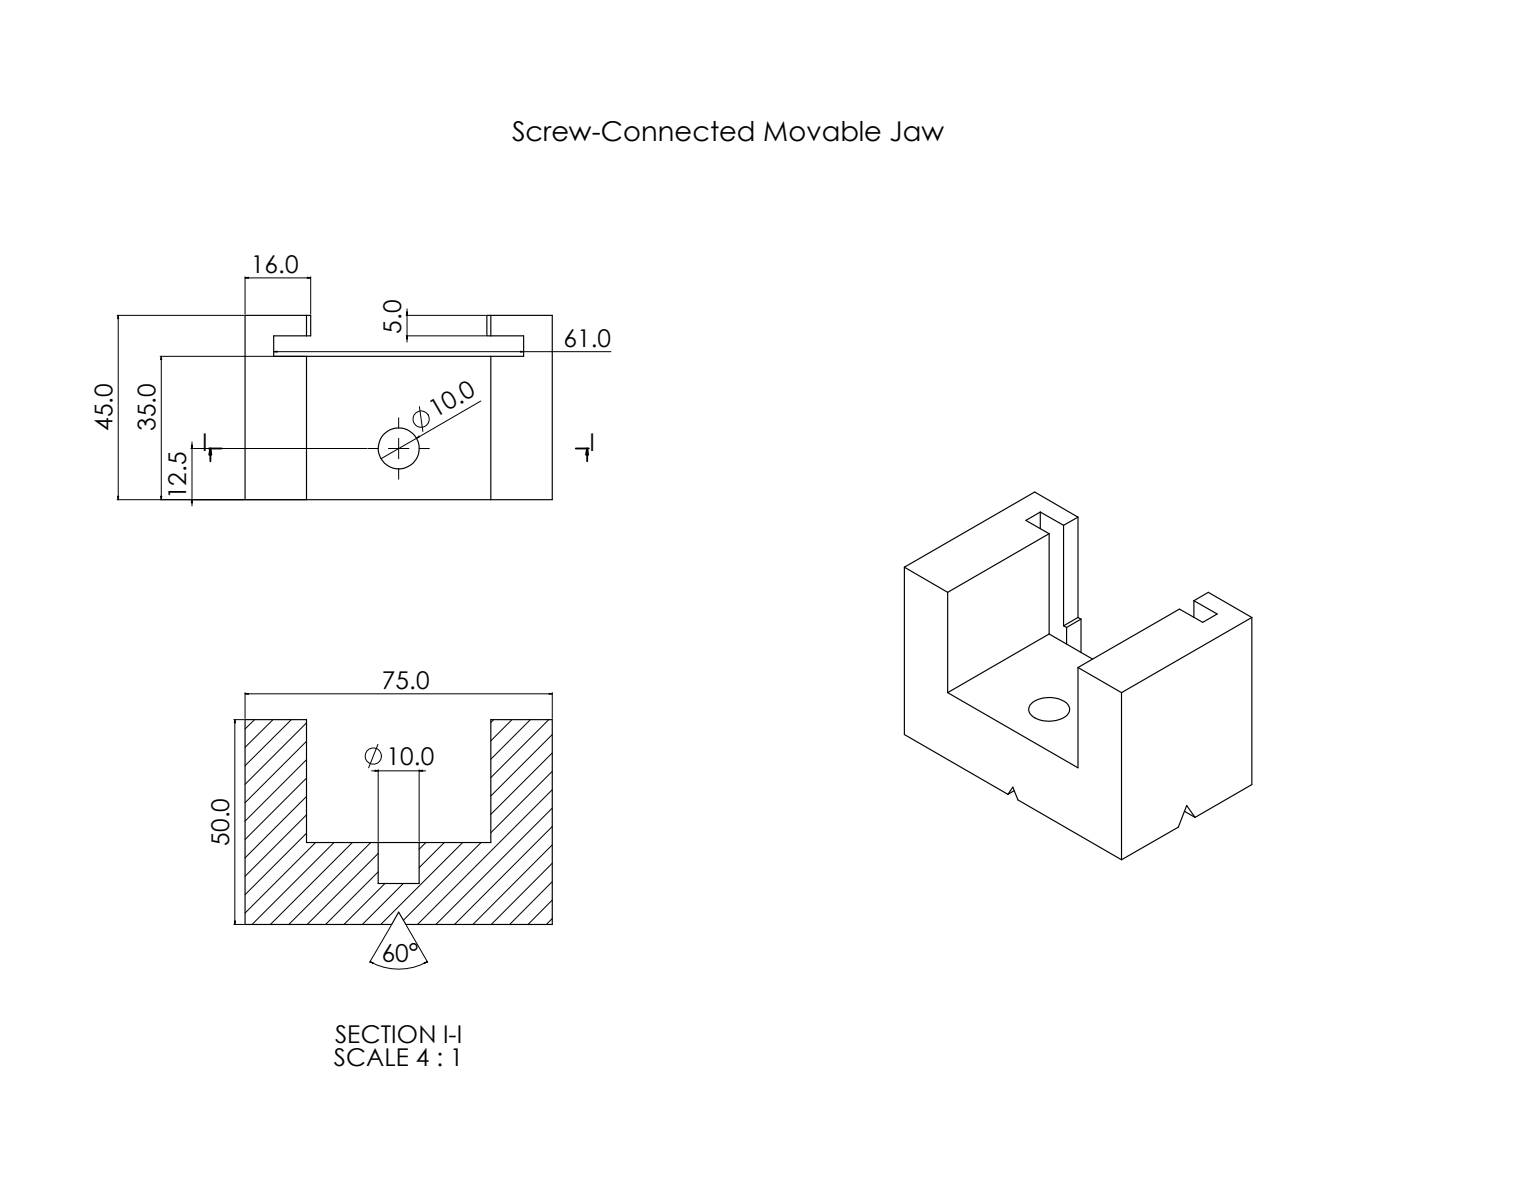
ISO-10303-21;
HEADER;
FILE_DESCRIPTION (('STEP AP214'),
    '1' );
FILE_NAME ('Screw-Connected Movable Jaw.step',
    '2026-10-24T22:31:37',
    ( '' ),
    ( '' ),
    'SwSTEP 2.0',
    'SolidWorks 2025',
    '' );
FILE_SCHEMA (( 'AUTOMOTIVE_DESIGN' ));
ENDSEC;

DATA;
#62=DIRECTION ( 'NONE',  ( 0.000000000000000000, -1.000000000000000000, 1.090355031989287297E-16 ) ) ;
#117=LINE ( 'NONE', #62385, #16927 ) ;
#143=CARTESIAN_POINT ( 'NONE',  ( -37.33262083840156009, 163.6868197944959888, -1.732050807568741524 ) ) ;
#194=ORIENTED_EDGE ( 'NONE', *, *, #7075, .T. ) ;
#425=EDGE_CURVE ( 'NONE', #74638, #6038, #70695, .T. ) ;
#505=DIRECTION ( 'NONE',  ( -0.8660254037844385966, -0.4999999999999999445, 5.782411586589351229E-17 ) ) ;
#555=DIRECTION ( 'NONE',  ( -0.8660254037844384856, -0.5000000000000002220, 5.782411586589354927E-17 ) ) ;
#594=ORIENTED_EDGE ( 'NONE', *, *, #77639, .T. ) ;
#731=ADVANCED_FACE ( 'NONE', ( #78063 ), #54223, .F. ) ;
#750=CARTESIAN_POINT ( 'NONE',  ( -17.69472717286124208, 126.6729902121449811, 2.598076211353400389 ) ) ;
#879=EDGE_CURVE ( 'NONE', #47755, #61485, #20257, .T. ) ;
#908=CARTESIAN_POINT ( 'NONE',  ( 5.968649350820379063, 188.6868197944959604, -22.49999999999984368 ) ) ;
#1042=ADVANCED_FACE ( 'NONE', ( #29840 ), #14643, .F. ) ;
#1055=DIRECTION ( 'NONE',  ( 3.817860598523670672E-18, 1.090355031989287297E-16, 1.000000000000000000 ) ) ;
#1129=ORIENTED_EDGE ( 'NONE', *, *, #70913, .F. ) ;
#1239=DIRECTION ( 'NONE',  ( 0.5000000000000004441, -0.8660254037844383745, -0.000000000000000000 ) ) ;
#1415=LINE ( 'NONE', #87069, #9047 ) ;
#1497=EDGE_LOOP ( 'NONE', ( #50090, #79860, #594, #87888 ) ) ;
#1639=EDGE_CURVE ( 'NONE', #18415, #51452, #44648, .T. ) ;
#2048=EDGE_CURVE ( 'NONE', #72912, #83865, #78409, .T. ) ;
#2098=ORIENTED_EDGE ( 'NONE', *, *, #49119, .T. ) ;
#2149=LINE ( 'NONE', #78150, #15677 ) ;
#2199=CLOSED_SHELL ( 'NONE', ( #75150, #7233, #84553, #37271, #22213, #44129, #61711, #25953, #74022, #4386, #1042, #68700, #27934, #56439, #64130, #11572, #38638, #98679, #79121, #731, #36244, #12582, #9749, #91004, #12653, #26400, #28305, #79766, #19607, #61517, #59063, #68707, #71578, #39382 ) ) ;
#2227=PRODUCT_DEFINITION_SHAPE ( 'NONE', 'NONE',  #80010 ) ;
#2485=ORIENTED_EDGE ( 'NONE', *, *, #31531, .F. ) ;
#2498=CARTESIAN_POINT ( 'NONE',  ( 5.968649350820482979, 188.6868197944959320, -37.49999999999994316 ) ) ;
#2564=ORIENTED_EDGE ( 'NONE', *, *, #90628, .T. ) ;
#2631=VECTOR ( 'NONE', #64054, 1000.000000000000000 ) ;
#2646=EDGE_CURVE ( 'NONE', #86838, #32226, #4151, .T. ) ;
#2647=CARTESIAN_POINT ( 'NONE',  ( -41.79694972978692391, 146.7012482093458914, -8.867527416774462878 ) ) ;
#2969=CARTESIAN_POINT ( 'NONE',  ( 2.487887237287232711, 134.7156766241960497, 22.50000000000002132 ) ) ;
#3041=VECTOR ( 'NONE', #9744, 1000.000000000000114 ) ;
#3155=ORIENTED_EDGE ( 'NONE', *, *, #18849, .T. ) ;
#3325=EDGE_LOOP ( 'NONE', ( #87906, #41347, #44835, #33520 ) ) ;
#3401=LINE ( 'NONE', #96620, #5789 ) ;
#3471=EDGE_CURVE ( 'NONE', #73274, #82623, #43663, .T. ) ;
#3574=CARTESIAN_POINT ( 'NONE',  ( -22.42236680055716036, 157.8615022471903444, 5.188172501216621122E-14 ) ) ;
#3633=CARTESIAN_POINT ( 'NONE',  ( -14.83262083840143575, 124.7156766241961208, 21.50000000000006750 ) ) ;
#3874=DIRECTION ( 'NONE',  ( -0.8660254037844384856, -0.5000000000000002220, -3.252519625699449945E-16 ) ) ;
#4014=LINE ( 'NONE', #33416, #90354 ) ;
#4047=LINE ( 'NONE', #87232, #75251 ) ;
#4062=ORIENTED_EDGE ( 'NONE', *, *, #77189, .T. ) ;
#4065=CARTESIAN_POINT ( 'NONE',  ( -14.83262083840142154, 124.7156766241961208, -37.49999999999995737 ) ) ;
#4151=LINE ( 'NONE', #80716, #24806 ) ;
#4181=CARTESIAN_POINT ( 'NONE',  ( -26.08262083840154233, 139.2012482093457493, 37.49999999999996447 ) ) ;
#4349=VERTEX_POINT ( 'NONE', #79754 ) ;
#4386=ADVANCED_FACE ( 'NONE', ( #59755 ), #36460, .F. ) ;
#4388=VECTOR ( 'NONE', #14547, 1000.000000000000000 ) ;
#4548=DIRECTION ( 'NONE',  ( -0.5000000000000003331, 0.8660254037844383745, 0.000000000000000000 ) ) ;
#4553=LINE ( 'NONE', #50644, #84057 ) ;
#4562=EDGE_CURVE ( 'NONE', #63766, #16186, #49551, .T. ) ;
#4738=FACE_OUTER_BOUND ( 'NONE', #58855, .T. ) ;
#4995=LINE ( 'NONE', #28269, #80233 ) ;
#5582=EDGE_CURVE ( 'NONE', #6163, #74234, #97394, .T. ) ;
#5666=VERTEX_POINT ( 'NONE', #10167 ) ;
#5677=ORIENTED_EDGE ( 'NONE', *, *, #59489, .F. ) ;
#5789=VECTOR ( 'NONE', #57061, 1000.000000000000000 ) ;
#5914=ORIENTED_EDGE ( 'NONE', *, *, #17435, .T. ) ;
#6038=VERTEX_POINT ( 'NONE', #64241 ) ;
#6163=VERTEX_POINT ( 'NONE', #89116 ) ;
#6186=VECTOR ( 'NONE', #3874, 1000.000000000000227 ) ;
#6215=EDGE_LOOP ( 'NONE', ( #59856, #62245, #86227, #58381 ) ) ;
#6329=CARTESIAN_POINT ( 'NONE',  ( -13.79761285583127872, 128.9229902121449811, 8.559299291603829198E-14 ) ) ;
#6632=VECTOR ( 'NONE', #76579, 1000.000000000000000 ) ;
#6865=DIRECTION ( 'NONE',  ( -2.168404344971021440E-16, 3.755786496842916807E-16, 1.000000000000000000 ) ) ;
#7006=VECTOR ( 'NONE', #78316, 1000.000000000000227 ) ;
#7075=EDGE_CURVE ( 'NONE', #88359, #90349, #41118, .T. ) ;
#7233=ADVANCED_FACE ( 'NONE', ( #82682 ), #51213, .F. ) ;
#7251=CARTESIAN_POINT ( 'NONE',  ( -17.33262083840142509, 129.0458036431182904, -30.52142883766501669 ) ) ;
#7266=CARTESIAN_POINT ( 'NONE',  ( -20.01211276271284945, 173.6868197944959036, -22.49999999999984013 ) ) ;
#7563=CARTESIAN_POINT ( 'NONE',  ( -19.83262083840137180, 133.3759306620404459, -30.52142883766495629 ) ) ;
#7571=SHAPE_REPRESENTATION ( 'Screw-Connected Movable Jaw', ( #68784 ), #31602 ) ;
#7578=VERTEX_POINT ( 'NONE', #71701 ) ;
#7683=CARTESIAN_POINT ( 'NONE',  ( -2.512112762712735314, 143.3759306620403891, -22.49999999999983658 ) ) ;
#7854=VECTOR ( 'NONE', #27344, 1000.000000000000000 ) ;
#7870=CARTESIAN_POINT ( 'NONE',  ( -37.33262083840156720, 163.6868197944959888, 1.732050807568908724 ) ) ;
#7916=DIRECTION ( 'NONE',  ( -0.5000000000000001110, 0.8660254037844384856, 0.000000000000000000 ) ) ;
#8114=LINE ( 'NONE', #22304, #30135 ) ;
#8168=ORIENTED_EDGE ( 'NONE', *, *, #19129, .T. ) ;
#8212=CARTESIAN_POINT ( 'NONE',  ( 28.46864935082050252, 149.7156766241961350, -37.49999999999994316 ) ) ;
#8322=VERTEX_POINT ( 'NONE', #70686 ) ;
#8363=PLANE ( 'NONE',  #70920 ) ;
#8478=EDGE_LOOP ( 'NONE', ( #51154, #77489, #24724, #33114, #10678, #81299 ) ) ;
#8670=EDGE_LOOP ( 'NONE', ( #87000, #21456, #59012, #82999, #14658, #48072, #24313, #5677 ) ) ;
#8671=ORIENTED_EDGE ( 'NONE', *, *, #77189, .F. ) ;
#8776=VERTEX_POINT ( 'NONE', #83914 ) ;
#8850=UNCERTAINTY_MEASURE_WITH_UNIT (LENGTH_MEASURE( 1.000000000000000082E-05 ), #27316, 'distance_accuracy_value', 'NONE');
#8993=CARTESIAN_POINT ( 'NONE',  ( -0.01211276271276783001, 139.0458036431182620, -22.49999999999983658 ) ) ;
#9045=ORIENTED_EDGE ( 'NONE', *, *, #14029, .T. ) ;
#9047=VECTOR ( 'NONE', #11022, 1000.000000000000000 ) ;
#9248=VECTOR ( 'NONE', #40481, 1000.000000000000114 ) ;
#9460=ORIENTED_EDGE ( 'NONE', *, *, #61819, .F. ) ;
#9580=CARTESIAN_POINT ( 'NONE',  ( -14.83262083840143575, 124.7156766241961208, -21.50000000000003197 ) ) ;
#9618=CARTESIAN_POINT ( 'NONE',  ( 19.98788723728717898, 104.4047874917408336, 22.50000000000002132 ) ) ;
#9744=DIRECTION ( 'NONE',  ( 0.5000000000000004441, -0.8660254037844383745, -0.000000000000000000 ) ) ;
#9749=ADVANCED_FACE ( 'NONE', ( #58583 ), #19135, .F. ) ;
#9823=CARTESIAN_POINT ( 'NONE',  ( 5.968649350820482979, 188.6868197944959320, -37.49999999999994316 ) ) ;
#9826=ORIENTED_EDGE ( 'NONE', *, *, #15394, .F. ) ;
#9889=ORIENTED_EDGE ( 'NONE', *, *, #15394, .T. ) ;
#9934=ORIENTED_EDGE ( 'NONE', *, *, #92492, .F. ) ;
#9947=EDGE_CURVE ( 'NONE', #12823, #82885, #37288, .T. ) ;
#9975=VECTOR ( 'NONE', #45768, 1000.000000000000000 ) ;
#9992=LINE ( 'NONE', #32770, #17278 ) ;
#10061=ORIENTED_EDGE ( 'NONE', *, *, #19856, .T. ) ;
#10167=CARTESIAN_POINT ( 'NONE',  ( -17.33262083840143930, 129.0458036431182904, 21.50000000000006750 ) ) ;
#10240=DIRECTION ( 'NONE',  ( -0.8944271909999158554, 0.000000000000000000, -0.4472135954999578722 ) ) ;
#10434=ORIENTED_EDGE ( 'NONE', *, *, #88822, .F. ) ;
#10616=ORIENTED_EDGE ( 'NONE', *, *, #56292, .F. ) ;
#10634=ORIENTED_EDGE ( 'NONE', *, *, #76967, .F. ) ;
#10642=LINE ( 'NONE', #71447, #37753 ) ;
#10678=ORIENTED_EDGE ( 'NONE', *, *, #71015, .T. ) ;
#10704=VECTOR ( 'NONE', #12962, 1000.000000000000227 ) ;
#10811=LINE ( 'NONE', #9823, #16722 ) ;
#10925=AXIS2_PLACEMENT_3D ( 'NONE', #55046, #78378, #18578 ) ;
#11022=DIRECTION ( 'NONE',  ( 0.8660254037844384856, 0.5000000000000002220, -5.782411586589354927E-17 ) ) ;
#11049=AXIS2_PLACEMENT_3D ( 'NONE', #65578, #50871, #42267 ) ;
#11078=CARTESIAN_POINT ( 'NONE',  ( 86.18027666378026197, 49.75620593066997799, 22.50000000000002842 ) ) ;
#11080=CARTESIAN_POINT ( 'NONE',  ( 42.87900647455834502, 24.75620593066997444, 1.732050807568941364 ) ) ;
#11087=CARTESIAN_POINT ( 'NONE',  ( 23.46864935082055581, 158.3759306620404743, -30.52142883766493853 ) ) ;
#11207=AXIS2_PLACEMENT_3D ( 'NONE', #41992, #58187, #72929 ) ;
#11363=ORIENTED_EDGE ( 'NONE', *, *, #96502, .F. ) ;
#11572=ADVANCED_FACE ( 'NONE', ( #50894 ), #27119, .F. ) ;
#11625=CARTESIAN_POINT ( 'NONE',  ( -11.26211276271278194, 158.5313752282681605, 5.249404841173988696E-14 ) ) ;
#11665=ORIENTED_EDGE ( 'NONE', *, *, #5582, .F. ) ;
#11880=PLANE ( 'NONE',  #54755 ) ;
#11930=PLANE ( 'NONE',  #43280 ) ;
#12162=FACE_OUTER_BOUND ( 'NONE', #51047, .T. ) ;
#12401=EDGE_CURVE ( 'NONE', #47755, #60445, #37275, .T. ) ;
#12582=ADVANCED_FACE ( 'NONE', ( #48381 ), #79325, .F. ) ;
#12653=ADVANCED_FACE ( 'NONE', ( #47118 ), #78039, .F. ) ;
#12667=CARTESIAN_POINT ( 'NONE',  ( -2.631798339875063064, 146.7012482093458914, -10.71504827818132277 ) ) ;
#12669=LINE ( 'NONE', #50636, #79981 ) ;
#12690=DIRECTION ( 'NONE',  ( 0.5000000000000004441, -0.8660254037844383745, -0.000000000000000000 ) ) ;
#12819=ORIENTED_EDGE ( 'NONE', *, *, #22660, .F. ) ;
#12823=VERTEX_POINT ( 'NONE', #96261 ) ;
#12846=CARTESIAN_POINT ( 'NONE',  ( -17.23454462704816947, 134.8759306620403038, 8.559299000364187034E-14 ) ) ;
#12962=DIRECTION ( 'NONE',  ( -0.8660254037844384856, -0.5000000000000002220, -3.252519625699449945E-16 ) ) ;
#13026=CARTESIAN_POINT ( 'NONE',  ( 25.96864935082048831, 154.0458036431183189, 30.52142883766506998 ) ) ;
#13092=VECTOR ( 'NONE', #72623, 1000.000000000000114 ) ;
#13113=FACE_OUTER_BOUND ( 'NONE', #15810, .T. ) ;
#13355=VECTOR ( 'NONE', #1239, 1000.000000000000114 ) ;
#13424=DIRECTION ( 'NONE',  ( 0.000000000000000000, 1.000000000000000000, 1.097929109219269329E-14 ) ) ;
#13577=FACE_OUTER_BOUND ( 'NONE', #6215, .T. ) ;
#13610=LINE ( 'NONE', #92150, #40083 ) ;
#13623=VECTOR ( 'NONE', #34224, 1000.000000000000114 ) ;
#13774=EDGE_LOOP ( 'NONE', ( #73707, #8671, #89866, #94192, #87422, #20562, #50702 ) ) ;
#13881=ORIENTED_EDGE ( 'NONE', *, *, #31531, .T. ) ;
#14029=EDGE_CURVE ( 'NONE', #61860, #89848, #10642, .T. ) ;
#14037=VECTOR ( 'NONE', #96964, 1000.000000000000227 ) ;
#14064=DIRECTION ( 'NONE',  ( -0.8944271909999158554, 0.000000000000000000, -0.4472135954999578722 ) ) ;
#14371=CARTESIAN_POINT ( 'NONE',  ( -21.75249381947928740, 146.7012482093458914, -37.49999999999995737 ) ) ;
#14434=DIRECTION ( 'NONE',  ( -0.5000000000000003331, 0.8660254037844383745, -9.251858538542982674E-17 ) ) ;
#14515=CARTESIAN_POINT ( 'NONE',  ( 86.18027666378027618, 49.75620593066998509, 1.003037947553365612E-13 ) ) ;
#14526=VERTEX_POINT ( 'NONE', #77303 ) ;
#14547=DIRECTION ( 'NONE',  ( -0.000000000000000000, -0.000000000000000000, 1.000000000000000000 ) ) ;
#14601=CARTESIAN_POINT ( 'NONE',  ( -13.79761285583127872, 128.9229902121449811, 8.559299291603829198E-14 ) ) ;
#14643=PLANE ( 'NONE',  #53793 ) ;
#14658=ORIENTED_EDGE ( 'NONE', *, *, #22404, .F. ) ;
#14688=ORIENTED_EDGE ( 'NONE', *, *, #42973, .F. ) ;
#15205=VERTEX_POINT ( 'NONE', #61955 ) ;
#15311=ORIENTED_EDGE ( 'NONE', *, *, #85316, .T. ) ;
#15354=CARTESIAN_POINT ( 'NONE',  ( 0.000000000000000000, 0.000000000000000000, 0.000000000000000000 ) ) ;
#15394=EDGE_CURVE ( 'NONE', #91009, #24841, #31779, .T. ) ;
#15543=ORIENTED_EDGE ( 'NONE', *, *, #53881, .F. ) ;
#15633=CARTESIAN_POINT ( 'NONE',  ( -21.75249381947928740, 146.7012482093458914, -48.95643923738973768 ) ) ;
#15677=VECTOR ( 'NONE', #32021, 1000.000000000000000 ) ;
#15689=DIRECTION ( 'NONE',  ( 0.8660254037844384856, 0.5000000000000002220, 0.000000000000000000 ) ) ;
#15810=EDGE_LOOP ( 'NONE', ( #17648, #1129, #54369, #36084 ) ) ;
#15951=CARTESIAN_POINT ( 'NONE',  ( 25.96864935082048831, 154.0458036431183189, 21.50000000000008527 ) ) ;
#16186=VERTEX_POINT ( 'NONE', #26218 ) ;
#16529=VERTEX_POINT ( 'NONE', #7266 ) ;
#16685=EDGE_CURVE ( 'NONE', #82885, #18415, #35514, .T. ) ;
#16722=VECTOR ( 'NONE', #65493, 1000.000000000000000 ) ;
#16908=EDGE_CURVE ( 'NONE', #6038, #8322, #9992, .T. ) ;
#16927=VECTOR ( 'NONE', #23898, 1000.000000000000227 ) ;
#17115=EDGE_CURVE ( 'NONE', #27140, #32226, #65792, .T. ) ;
#17141=VERTEX_POINT ( 'NONE', #37257 ) ;
#17278=VECTOR ( 'NONE', #31755, 999.9999999999998863 ) ;
#17419=CARTESIAN_POINT ( 'NONE',  ( -37.33262083840143930, 163.6868197944959036, -37.49999999999995737 ) ) ;
#17422=CARTESIAN_POINT ( 'NONE',  ( 5.968649350820482979, 188.6868197944959320, -37.49999999999994316 ) ) ;
#17430=ORIENTED_EDGE ( 'NONE', *, *, #98473, .F. ) ;
#17435=EDGE_CURVE ( 'NONE', #5666, #82885, #2149, .T. ) ;
#17498=VERTEX_POINT ( 'NONE', #143 ) ;
#17537=VECTOR ( 'NONE', #29031, 999.9999999999998863 ) ;
#17648=ORIENTED_EDGE ( 'NONE', *, *, #85806, .T. ) ;
#17687=VERTEX_POINT ( 'NONE', #82679 ) ;
#17710=LINE ( 'NONE', #25295, #28391 ) ;
#17920=ORIENTED_EDGE ( 'NONE', *, *, #85209, .T. ) ;
#17929=ORIENTED_EDGE ( 'NONE', *, *, #45726, .T. ) ;
#17990=DIRECTION ( 'NONE',  ( 0.000000000000000000, -1.000000000000000000, 1.090355031989287297E-16 ) ) ;
#18047=ORIENTED_EDGE ( 'NONE', *, *, #88822, .T. ) ;
#18131=CARTESIAN_POINT ( 'NONE',  ( 5.968649350820472321, 188.6868197944958752, 22.50000000000001421 ) ) ;
#18261=EDGE_CURVE ( 'NONE', #48830, #17141, #80171, .T. ) ;
#18415=VERTEX_POINT ( 'NONE', #83535 ) ;
#18479=CARTESIAN_POINT ( 'NONE',  ( 28.46864935082048831, 149.7156766241961350, -21.50000000000001421 ) ) ;
#18536=CARTESIAN_POINT ( 'NONE',  ( 2.487887237287232711, 134.7156766241960497, 21.50000000000007461 ) ) ;
#18571=CARTESIAN_POINT ( 'NONE',  ( 2.487887237287232711, 134.7156766241960497, -22.49999999999983302 ) ) ;
#18578=DIRECTION ( 'NONE',  ( 0.5000000000000003331, -0.8660254037844383745, 0.000000000000000000 ) ) ;
#18634=CARTESIAN_POINT ( 'NONE',  ( -2.512112762712737091, 143.3759306620403891, -30.52142883766493853 ) ) ;
#18664=DIRECTION ( 'NONE',  ( -2.816764622163176999E-16, -1.626259812849725466E-16, 1.000000000000000000 ) ) ;
#18849=EDGE_CURVE ( 'NONE', #65623, #88359, #32544, .T. ) ;
#18903=FACE_OUTER_BOUND ( 'NONE', #1497, .T. ) ;
#19036=( GEOMETRIC_REPRESENTATION_CONTEXT ( 3 ) GLOBAL_UNCERTAINTY_ASSIGNED_CONTEXT ( ( #8850 ) ) GLOBAL_UNIT_ASSIGNED_CONTEXT ( ( #27316, #62931, #40116 ) ) REPRESENTATION_CONTEXT ( 'NONE', 'WORKASPACE' ) );
#19049=ORIENTED_EDGE ( 'NONE', *, *, #91374, .F. ) ;
#19129=EDGE_CURVE ( 'NONE', #31218, #65623, #68910, .T. ) ;
#19135=PLANE ( 'NONE',  #98371 ) ;
#19240=VECTOR ( 'NONE', #80991, 1000.000000000000000 ) ;
#19341=CARTESIAN_POINT ( 'NONE',  ( 86.18027666378026197, 49.75620593066997799, 22.50000000000002842 ) ) ;
#19380=AXIS2_PLACEMENT_3D ( 'NONE', #15951, #39721, #77776 ) ;
#19520=AXIS2_PLACEMENT_3D ( 'NONE', #27495, #50765, #58364 ) ;
#19582=PLANE ( 'NONE',  #49676 ) ;
#19607=ADVANCED_FACE ( 'NONE', ( #97729 ), #43986, .F. ) ;
#19629=EDGE_CURVE ( 'NONE', #63672, #16186, #1415, .T. ) ;
#19772=VECTOR ( 'NONE', #58847, 1000.000000000000114 ) ;
#19856=EDGE_CURVE ( 'NONE', #48417, #92799, #90032, .T. ) ;
#19998=VECTOR ( 'NONE', #80244, 1000.000000000000000 ) ;
#20055=DIRECTION ( 'NONE',  ( -1.000000000000000000, 0.000000000000000000, -2.816764622163176999E-16 ) ) ;
#20145=VERTEX_POINT ( 'NONE', #14371 ) ;
#20257=LINE ( 'NONE', #12667, #24876 ) ;
#20298=DIRECTION ( 'NONE',  ( 0.8660254037844385966, 0.5000000000000002220, 7.511572993685832627E-16 ) ) ;
#20423=ORIENTED_EDGE ( 'NONE', *, *, #20676, .F. ) ;
#20510=EDGE_LOOP ( 'NONE', ( #12819, #50067, #64992, #25275, #70880, #10061 ) ) ;
#20548=ORIENTED_EDGE ( 'NONE', *, *, #88172, .F. ) ;
#20562=ORIENTED_EDGE ( 'NONE', *, *, #39641, .F. ) ;
#20676=EDGE_CURVE ( 'NONE', #12823, #89585, #37230, .T. ) ;
#20793=VECTOR ( 'NONE', #95392, 1000.000000000000114 ) ;
#20803=CARTESIAN_POINT ( 'NONE',  ( 42.87900647455834502, 24.75620593066997444, 8.404119662683931360E-14 ) ) ;
#20833=DIRECTION ( 'NONE',  ( 8.673617379884076887E-16, 0.000000000000000000, -1.000000000000000000 ) ) ;
#21031=CARTESIAN_POINT ( 'NONE',  ( 25.96864935082050252, 154.0458036431183189, -30.52142883766499892 ) ) ;
#21035=AXIS2_PLACEMENT_3D ( 'NONE', #73746, #88011, #20055 ) ;
#21094=ORIENTED_EDGE ( 'NONE', *, *, #24594, .F. ) ;
#21167=DIRECTION ( 'NONE',  ( -0.8660254037844384856, -0.5000000000000002220, -3.252519625699449945E-16 ) ) ;
#21213=EDGE_CURVE ( 'NONE', #63766, #7578, #97327, .T. ) ;
#21281=DIRECTION ( 'NONE',  ( -0.5000000000000003331, 0.8660254037844385966, -4.336808689942041895E-16 ) ) ;
#21288=ORIENTED_EDGE ( 'NONE', *, *, #35737, .F. ) ;
#21324=EDGE_CURVE ( 'NONE', #70724, #90349, #4995, .T. ) ;
#21441=DIRECTION ( 'NONE',  ( -0.5000000000000003331, 0.8660254037844383745, -5.669937756276021476E-31 ) ) ;
#21456=ORIENTED_EDGE ( 'NONE', *, *, #50443, .T. ) ;
#21615=EDGE_LOOP ( 'NONE', ( #27858, #70387, #9826, #71355, #88499, #20548, #88494, #35459, #44301, #10616, #18047 ) ) ;
#21737=CARTESIAN_POINT ( 'NONE',  ( 25.96864935082050252, 154.0458036431183189, -21.50000000000001421 ) ) ;
#21741=DIRECTION ( 'NONE',  ( 1.000000000000000000, 0.000000000000000000, 2.816764622163176999E-16 ) ) ;
#21771=VERTEX_POINT ( 'NONE', #30148 ) ;
#21895=ORIENTED_EDGE ( 'NONE', *, *, #85316, .F. ) ;
#22027=DIRECTION ( 'NONE',  ( -0.4999999999999995004, 0.8660254037844389297, -1.249000902703319567E-14 ) ) ;
#22038=AXIS2_PLACEMENT_3D ( 'NONE', #74426, #88665, #73414 ) ;
#22040=EDGE_CURVE ( 'NONE', #89848, #16529, #8114, .T. ) ;
#22209=DIRECTION ( 'NONE',  ( -0.8660254037844384856, -0.5000000000000002220, 0.000000000000000000 ) ) ;
#22213=ADVANCED_FACE ( 'NONE', ( #34402 ), #90135, .T. ) ;
#22246=DIRECTION ( 'NONE',  ( -0.8660254037844384856, -0.5000000000000002220, -3.252519625699449945E-16 ) ) ;
#22304=CARTESIAN_POINT ( 'NONE',  ( 31.94941146435350987, 203.6868197944959320, -22.49999999999984368 ) ) ;
#22320=CIRCLE ( 'NONE', #95202, 4.999999999999993783 ) ;
#22347=EDGE_CURVE ( 'NONE', #49527, #70724, #55562, .T. ) ;
#22361=LINE ( 'NONE', #75088, #76135 ) ;
#22365=DIRECTION ( 'NONE',  ( 4.546899780356473057E-16, -0.000000000000000000, -1.000000000000000000 ) ) ;
#22404=EDGE_CURVE ( 'NONE', #90349, #6038, #22768, .T. ) ;
#22660=EDGE_CURVE ( 'NONE', #27862, #92799, #37221, .T. ) ;
#22768=LINE ( 'NONE', #9580, #86824 ) ;
#23037=DIRECTION ( 'NONE',  ( 0.8660254037844385966, 0.5000000000000004441, 0.000000000000000000 ) ) ;
#23066=ORIENTED_EDGE ( 'NONE', *, *, #96502, .T. ) ;
#23177=LINE ( 'NONE', #14601, #41431 ) ;
#23237=CARTESIAN_POINT ( 'NONE',  ( -24.06189489623784183, 146.7012482093458914, 8.087813781312181686E-14 ) ) ;
#23288=FACE_OUTER_BOUND ( 'NONE', #82900, .T. ) ;
#23457=DIRECTION ( 'NONE',  ( 1.000000000000000000, 0.000000000000000000, 0.000000000000000000 ) ) ;
#23898=DIRECTION ( 'NONE',  ( -0.5000000000000001110, 0.8660254037844384856, 2.775557561562890427E-17 ) ) ;
#23936=EDGE_CURVE ( 'NONE', #6163, #47559, #49559, .T. ) ;
#24052=DIRECTION ( 'NONE',  ( 0.8944271909999157444, 0.000000000000000000, -0.4472135954999582608 ) ) ;
#24313=ORIENTED_EDGE ( 'NONE', *, *, #53158, .F. ) ;
#24594=EDGE_CURVE ( 'NONE', #49426, #89848, #95977, .T. ) ;
#24724=ORIENTED_EDGE ( 'NONE', *, *, #70913, .T. ) ;
#24785=LINE ( 'NONE', #9618, #9248 ) ;
#24806=VECTOR ( 'NONE', #51240, 1000.000000000000227 ) ;
#24819=CARTESIAN_POINT ( 'NONE',  ( 19.98788723728717898, 104.4047874917408336, 22.50000000000002132 ) ) ;
#24841=VERTEX_POINT ( 'NONE', #12846 ) ;
#24845=DIRECTION ( 'NONE',  ( 0.8660254037844383745, 0.5000000000000003331, -0.000000000000000000 ) ) ;
#24876=VECTOR ( 'NONE', #71965, 1000.000000000000227 ) ;
#24910=EDGE_CURVE ( 'NONE', #86838, #81759, #80224, .T. ) ;
#24966=ORIENTED_EDGE ( 'NONE', *, *, #61819, .T. ) ;
#24983=LINE ( 'NONE', #55369, #13092 ) ;
#25087=ORIENTED_EDGE ( 'NONE', *, *, #53881, .T. ) ;
#25091=ORIENTED_EDGE ( 'NONE', *, *, #4562, .F. ) ;
#25122=ORIENTED_EDGE ( 'NONE', *, *, #38764, .T. ) ;
#25275=ORIENTED_EDGE ( 'NONE', *, *, #94948, .F. ) ;
#25295=CARTESIAN_POINT ( 'NONE',  ( -37.33262083840143930, 163.6868197944959036, -37.49999999999995737 ) ) ;
#25325=DIRECTION ( 'NONE',  ( -0.5000000000000002220, 0.8660254037844385966, -9.251858538542986372E-17 ) ) ;
#25369=ORIENTED_EDGE ( 'NONE', *, *, #33162, .F. ) ;
#25425=VECTOR ( 'NONE', #76179, 1000.000000000000000 ) ;
#25667=LINE ( 'NONE', #56027, #91730 ) ;
#25699=CARTESIAN_POINT ( 'NONE',  ( 25.96864935082050252, 154.0458036431183189, -21.50000000000001421 ) ) ;
#25799=DIRECTION ( 'NONE',  ( -0.8660254037844384856, -0.5000000000000002220, -3.252519625699449945E-16 ) ) ;
#25834=EDGE_CURVE ( 'NONE', #31218, #74638, #45101, .T. ) ;
#25953=ADVANCED_FACE ( 'NONE', ( #23288 ), #70395, .F. ) ;
#26128=LINE ( 'NONE', #18536, #13623 ) ;
#26131=EDGE_CURVE ( 'NONE', #48830, #83821, #17710, .T. ) ;
#26218=CARTESIAN_POINT ( 'NONE',  ( 28.46864935082042081, 149.7156766241961066, 22.50000000000001776 ) ) ;
#26394=ORIENTED_EDGE ( 'NONE', *, *, #879, .F. ) ;
#26400=ADVANCED_FACE ( 'NONE', ( #13113 ), #36379, .F. ) ;
#26429=CARTESIAN_POINT ( 'NONE',  ( -14.83262083840143575, 124.7156766241961208, -21.50000000000003197 ) ) ;
#26539=DIRECTION ( 'NONE',  ( -1.850371707708595795E-16, -7.401486830834383181E-16, 1.000000000000000000 ) ) ;
#26574=DIRECTION ( 'NONE',  ( -1.000000000000000000, 0.000000000000000000, -2.816764622163179958E-16 ) ) ;
#26667=ORIENTED_EDGE ( 'NONE', *, *, #2048, .T. ) ;
#26902=ORIENTED_EDGE ( 'NONE', *, *, #22040, .T. ) ;
#27053=DIRECTION ( 'NONE',  ( 0.000000000000000000, -1.000000000000000000, 1.065403912962273439E-14 ) ) ;
#27060=DIRECTION ( 'NONE',  ( -0.000000000000000000, -0.000000000000000000, 1.000000000000000000 ) ) ;
#27083=DIRECTION ( 'NONE',  ( 3.817860598523670672E-18, 1.090355031989287297E-16, 1.000000000000000000 ) ) ;
#27119=PLANE ( 'NONE',  #30732 ) ;
#27140=VERTEX_POINT ( 'NONE', #34862 ) ;
#27277=ORIENTED_EDGE ( 'NONE', *, *, #3471, .T. ) ;
#27285=AXIS2_PLACEMENT_3D ( 'NONE', #29920, #83159, #45115 ) ;
#27316=( LENGTH_UNIT ( ) NAMED_UNIT ( * ) SI_UNIT ( .MILLI., .METRE. ) );
#27344=DIRECTION ( 'NONE',  ( -8.673617379884075901E-16, 0.000000000000000000, 1.000000000000000000 ) ) ;
#27446=CARTESIAN_POINT ( 'NONE',  ( 28.46864935082048831, 149.7156766241961350, -21.50000000000001421 ) ) ;
#27495=CARTESIAN_POINT ( 'NONE',  ( -22.42236680055716036, 157.8615022471903444, 5.188172501216621122E-14 ) ) ;
#27500=CARTESIAN_POINT ( 'NONE',  ( 2.487887237287232711, 134.7156766241960497, -21.50000000000002487 ) ) ;
#27579=DIRECTION ( 'NONE',  ( 2.816764622163179958E-16, 1.626259812849721275E-16, -1.000000000000000000 ) ) ;
#27599=PLANE ( 'NONE',  #11049 ) ;
#27753=ORIENTED_EDGE ( 'NONE', *, *, #39641, .T. ) ;
#27858=ORIENTED_EDGE ( 'NONE', *, *, #1639, .T. ) ;
#27862=VERTEX_POINT ( 'NONE', #96988 ) ;
#27910=CARTESIAN_POINT ( 'NONE',  ( 28.46864935082048831, 149.7156766241961350, -21.50000000000001421 ) ) ;
#27934=ADVANCED_FACE ( 'NONE', ( #95509 ), #56930, .F. ) ;
#28098=DIRECTION ( 'NONE',  ( 0.8660254037844384856, 0.5000000000000002220, 0.000000000000000000 ) ) ;
#28110=CYLINDRICAL_SURFACE ( 'NONE', #33385, 4.999999999999993783 ) ;
#28269=CARTESIAN_POINT ( 'NONE',  ( -14.83262083840143575, 124.7156766241961208, -21.50000000000003197 ) ) ;
#28304=DIRECTION ( 'NONE',  ( -0.5000000000000003331, 0.8660254037844385966, -4.336808689942039923E-16 ) ) ;
#28305=ADVANCED_FACE ( 'NONE', ( #89954 ), #28110, .F. ) ;
#28332=CARTESIAN_POINT ( 'NONE',  ( -17.33262083840142509, 129.0458036431182904, -21.50000000000003197 ) ) ;
#28377=PLANE ( 'NONE',  #56382 ) ;
#28391=VECTOR ( 'NONE', #79551, 1000.000000000000000 ) ;
#28459=DIRECTION ( 'NONE',  ( 0.4999999999999973910, -0.8660254037844401509, -1.249000902703321145E-14 ) ) ;
#28505=ORIENTED_EDGE ( 'NONE', *, *, #50988, .T. ) ;
#28535=VECTOR ( 'NONE', #34146, 1000.000000000000227 ) ;
#28689=CARTESIAN_POINT ( 'NONE',  ( -14.83262083840143575, 124.7156766241961208, 21.50000000000006750 ) ) ;
#28765=PLANE ( 'NONE',  #94887 ) ;
#28808=DIRECTION ( 'NONE',  ( -0.4999999999999995004, -0.8660254037844389297, -2.816764622163176506E-16 ) ) ;
#28925=CARTESIAN_POINT ( 'NONE',  ( -17.33262083840143930, 129.0458036431182904, 30.52142883766505221 ) ) ;
#29009=PRODUCT ( 'Screw-Connected Movable Jaw', 'Screw-Connected Movable Jaw', '', ( #65967 ) ) ;
#29031=DIRECTION ( 'NONE',  ( -0.5000000000000002220, 0.8660254037844385966, 0.000000000000000000 ) ) ;
#29059=ORIENTED_EDGE ( 'NONE', *, *, #45821, .T. ) ;
#29066=VECTOR ( 'NONE', #81499, 1000.000000000000000 ) ;
#29112=LINE ( 'NONE', #64233, #66139 ) ;
#29179=APPLICATION_CONTEXT ( 'automotive_design' ) ;
#29253=DIRECTION ( 'NONE',  ( -0.5000000000000002220, 0.8660254037844385966, -9.251858538542986372E-17 ) ) ;
#29314=LINE ( 'NONE', #50598, #80672 ) ;
#29350=CARTESIAN_POINT ( 'NONE',  ( 28.46864935082048831, 149.7156766241961350, 21.50000000000008527 ) ) ;
#29395=ORIENTED_EDGE ( 'NONE', *, *, #59489, .T. ) ;
#29488=ORIENTED_EDGE ( 'NONE', *, *, #16685, .F. ) ;
#29708=PLANE ( 'NONE',  #76816 ) ;
#29840=FACE_OUTER_BOUND ( 'NONE', #45774, .T. ) ;
#29920=CARTESIAN_POINT ( 'NONE',  ( 42.87900647455834502, 24.75620593066997444, 8.404119662683931360E-14 ) ) ;
#30040=CARTESIAN_POINT ( 'NONE',  ( 25.96864935082048831, 154.0458036431183189, 21.50000000000008527 ) ) ;
#30135=VECTOR ( 'NONE', #505, 1000.000000000000114 ) ;
#30146=FACE_OUTER_BOUND ( 'NONE', #32259, .T. ) ;
#30148=CARTESIAN_POINT ( 'NONE',  ( 25.96864935082043857, 154.0458036431183473, -22.49999999999983658 ) ) ;
#30284=DIRECTION ( 'NONE',  ( -3.817860598523670672E-18, -1.090355031989287297E-16, -1.000000000000000000 ) ) ;
#30424=ORIENTED_EDGE ( 'NONE', *, *, #90628, .F. ) ;
#30491=EDGE_CURVE ( 'NONE', #38493, #60445, #99467, .T. ) ;
#30732=AXIS2_PLACEMENT_3D ( 'NONE', #64615, #88984, #28098 ) ;
#30769=ORIENTED_EDGE ( 'NONE', *, *, #85209, .F. ) ;
#31218=VERTEX_POINT ( 'NONE', #83136 ) ;
#31531=EDGE_CURVE ( 'NONE', #88359, #49527, #59922, .T. ) ;
#31602=( GEOMETRIC_REPRESENTATION_CONTEXT ( 3 ) GLOBAL_UNCERTAINTY_ASSIGNED_CONTEXT ( ( #55426 ) ) GLOBAL_UNIT_ASSIGNED_CONTEXT ( ( #56367, #57864, #51251 ) ) REPRESENTATION_CONTEXT ( 'NONE', 'WORKASPACE' ) );
#31653=DIRECTION ( 'NONE',  ( -0.7499999999999993339, -0.4330127018922203530, -0.4999999999999999445 ) ) ;
#31661=ORIENTED_EDGE ( 'NONE', *, *, #7075, .F. ) ;
#31750=EDGE_LOOP ( 'NONE', ( #44607, #47418, #87963, #5914, #46934, #91670 ) ) ;
#31755=DIRECTION ( 'NONE',  ( -0.5000000000000002220, 0.8660254037844385966, 0.000000000000000000 ) ) ;
#31778=EDGE_CURVE ( 'NONE', #61485, #97002, #87311, .T. ) ;
#31779=LINE ( 'NONE', #78415, #94502 ) ;
#31831=CARTESIAN_POINT ( 'NONE',  ( 23.46864935082052739, 158.3759306620404743, 30.52142883766500603 ) ) ;
#31983=DIRECTION ( 'NONE',  ( 4.546899780356473057E-16, -0.000000000000000000, -1.000000000000000000 ) ) ;
#32021=DIRECTION ( 'NONE',  ( 0.000000000000000000, 0.000000000000000000, 1.000000000000000000 ) ) ;
#32147=FACE_OUTER_BOUND ( 'NONE', #55731, .T. ) ;
#32226=VERTEX_POINT ( 'NONE', #11625 ) ;
#32259=EDGE_LOOP ( 'NONE', ( #52528, #94238, #44454, #86918 ) ) ;
#32278=DIRECTION ( 'NONE',  ( -0.8660254037844384856, -0.5000000000000002220, -3.252519625699449945E-16 ) ) ;
#32286=EDGE_CURVE ( 'NONE', #65623, #71581, #13610, .T. ) ;
#32452=ORIENTED_EDGE ( 'NONE', *, *, #16685, .T. ) ;
#32544=LINE ( 'NONE', #83918, #53170 ) ;
#32591=CARTESIAN_POINT ( 'NONE',  ( -24.63924516542739696, 141.7012482093459198, 1.426039447152360146E-13 ) ) ;
#32770=CARTESIAN_POINT ( 'NONE',  ( -14.83262083840142154, 124.7156766241961208, -37.49999999999995737 ) ) ;
#33017=EDGE_LOOP ( 'NONE', ( #31661, #13881, #85607, #69698 ) ) ;
#33114=ORIENTED_EDGE ( 'NONE', *, *, #70740, .F. ) ;
#33120=CARTESIAN_POINT ( 'NONE',  ( 25.96864935082050252, 154.0458036431183189, -30.52142883766499892 ) ) ;
#33124=ORIENTED_EDGE ( 'NONE', *, *, #3471, .F. ) ;
#33162=EDGE_CURVE ( 'NONE', #14526, #48417, #81409, .T. ) ;
#33176=LINE ( 'NONE', #55449, #40226 ) ;
#33385=AXIS2_PLACEMENT_3D ( 'NONE', #89000, #43803, #65612 ) ;
#33416=CARTESIAN_POINT ( 'NONE',  ( 2.487887237287232711, 134.7156766241960497, 21.50000000000008527 ) ) ;
#33520=ORIENTED_EDGE ( 'NONE', *, *, #19629, .F. ) ;
#33609=LINE ( 'NONE', #57389, #19998 ) ;
#33638=VECTOR ( 'NONE', #22246, 1000.000000000000227 ) ;
#33707=VECTOR ( 'NONE', #55893, 1000.000000000000000 ) ;
#33779=CARTESIAN_POINT ( 'NONE',  ( 23.46864935082055581, 158.3759306620404743, -30.52142883766493853 ) ) ;
#33846=DIRECTION ( 'NONE',  ( 0.8660254037844385966, 0.4999999999999999445, -5.782411586589351229E-17 ) ) ;
#33895=EDGE_LOOP ( 'NONE', ( #84934, #67380, #98125, #48550 ) ) ;
#34109=DIRECTION ( 'NONE',  ( 0.4999999999999995004, 0.8660254037844389297, 0.000000000000000000 ) ) ;
#34146=DIRECTION ( 'NONE',  ( 0.4999999999999973910, -0.8660254037844401509, -1.249000902703321145E-14 ) ) ;
#34224=DIRECTION ( 'NONE',  ( 0.5000000000000003331, -0.8660254037844384856, -2.218671295934096141E-31 ) ) ;
#34308=DIRECTION ( 'NONE',  ( -3.817860598523670672E-18, -1.090355031989287297E-16, -1.000000000000000000 ) ) ;
#34402=FACE_OUTER_BOUND ( 'NONE', #87386, .T. ) ;
#34733=FACE_OUTER_BOUND ( 'NONE', #62075, .T. ) ;
#34862=CARTESIAN_POINT ( 'NONE',  ( -16.26211276271277839, 167.1916292661125283, 5.188172501216621122E-14 ) ) ;
#35020=DIRECTION ( 'NONE',  ( -0.8660254037844384856, -0.5000000000000002220, -3.252519625699449945E-16 ) ) ;
#35453=DIRECTION ( 'NONE',  ( 0.000000000000000000, 0.000000000000000000, -1.000000000000000000 ) ) ;
#35459=ORIENTED_EDGE ( 'NONE', *, *, #62771, .T. ) ;
#35514=LINE ( 'NONE', #28925, #55444 ) ;
#35695=ORIENTED_EDGE ( 'NONE', *, *, #84144, .T. ) ;
#35737=EDGE_CURVE ( 'NONE', #57299, #14526, #95383, .T. ) ;
#35769=EDGE_LOOP ( 'NONE', ( #40952, #98293, #2485, #66969 ) ) ;
#35822=ORIENTED_EDGE ( 'NONE', *, *, #18261, .T. ) ;
#35825=ORIENTED_EDGE ( 'NONE', *, *, #17435, .F. ) ;
#35841=CARTESIAN_POINT ( 'NONE',  ( -20.01211276271284945, 173.6868197944959036, 22.50000000000001421 ) ) ;
#36084=ORIENTED_EDGE ( 'NONE', *, *, #19129, .F. ) ;
#36187=CARTESIAN_POINT ( 'NONE',  ( 25.96864935082050252, 154.0458036431183189, -22.49999999999984013 ) ) ;
#36196=EDGE_CURVE ( 'NONE', #81759, #86838, #50011, .T. ) ;
#36239=VECTOR ( 'NONE', #21167, 1000.000000000000227 ) ;
#36244=ADVANCED_FACE ( 'NONE', ( #81532 ), #57682, .F. ) ;
#36284=DIRECTION ( 'NONE',  ( 8.673617379884080832E-16, -0.000000000000000000, -1.000000000000000000 ) ) ;
#36351=ORIENTED_EDGE ( 'NONE', *, *, #62771, .F. ) ;
#36379=PLANE ( 'NONE',  #36553 ) ;
#36460=PLANE ( 'NONE',  #37517 ) ;
#36553=AXIS2_PLACEMENT_3D ( 'NONE', #67283, #30284, #46983 ) ;
#36637=CARTESIAN_POINT ( 'NONE',  ( -15.65624769481498468, 157.2602562327093381, -7.250946663043509766 ) ) ;
#36701=AXIS2_PLACEMENT_3D ( 'NONE', #15633, #93180, #100268 ) ;
#36951=VECTOR ( 'NONE', #35020, 1000.000000000000227 ) ;
#37065=ORIENTED_EDGE ( 'NONE', *, *, #18261, .F. ) ;
#37144=DIRECTION ( 'NONE',  ( 0.000000000000000000, 0.000000000000000000, 1.000000000000000000 ) ) ;
#37221=LINE ( 'NONE', #59004, #10704 ) ;
#37230=LINE ( 'NONE', #74280, #42914 ) ;
#37247=PLANE ( 'NONE',  #63251 ) ;
#37257=CARTESIAN_POINT ( 'NONE',  ( -34.73454462704830803, 165.1868197944959036, 8.171888229646977204E-14 ) ) ;
#37271=ADVANCED_FACE ( 'NONE', ( #97990 ), #27599, .F. ) ;
#37275=LINE ( 'NONE', #90026, #46921 ) ;
#37288=LINE ( 'NONE', #13026, #64371 ) ;
#37406=LINE ( 'NONE', #92656, #81987 ) ;
#37436=ORIENTED_EDGE ( 'NONE', *, *, #45821, .F. ) ;
#37517=AXIS2_PLACEMENT_3D ( 'NONE', #98289, #21281, #89245 ) ;
#37753=VECTOR ( 'NONE', #25325, 999.9999999999998863 ) ;
#38037=DIRECTION ( 'NONE',  ( 0.000000000000000000, 0.000000000000000000, -1.000000000000000000 ) ) ;
#38493=VERTEX_POINT ( 'NONE', #68162 ) ;
#38561=VECTOR ( 'NONE', #37144, 1000.000000000000000 ) ;
#38638=ADVANCED_FACE ( 'NONE', ( #81309 ), #11880, .F. ) ;
#38764=EDGE_CURVE ( 'NONE', #63766, #12823, #68539, .T. ) ;
#38936=PLANE ( 'NONE',  #36701 ) ;
#39264=VECTOR ( 'NONE', #81458, 1000.000000000000000 ) ;
#39382=ADVANCED_FACE ( 'NONE', ( #4738 ), #49829, .F. ) ;
#39489=CARTESIAN_POINT ( 'NONE',  ( -0.01211276271276175848, 139.0458036431182620, -21.50000000000002487 ) ) ;
#39555=EDGE_LOOP ( 'NONE', ( #29395, #92833, #11665, #74989 ) ) ;
#39641=EDGE_CURVE ( 'NONE', #74638, #49426, #99924, .T. ) ;
#39699=CARTESIAN_POINT ( 'NONE',  ( -14.83262083840144996, 124.7156766241961208, 37.49999999999998579 ) ) ;
#39718=LINE ( 'NONE', #63546, #2631 ) ;
#39721=DIRECTION ( 'NONE',  ( 0.5000000000000003331, -0.8660254037844385966, 0.000000000000000000 ) ) ;
#40083=VECTOR ( 'NONE', #67291, 1000.000000000000114 ) ;
#40116=( NAMED_UNIT ( * ) SI_UNIT ( $, .STERADIAN. ) SOLID_ANGLE_UNIT ( ) );
#40226=VECTOR ( 'NONE', #31653, 1000.000000000000114 ) ;
#40481=DIRECTION ( 'NONE',  ( -0.5000000000000003331, 0.8660254037844383745, -9.251858538542983907E-17 ) ) ;
#40504=CARTESIAN_POINT ( 'NONE',  ( -21.75249381947928740, 146.7012482093458914, 37.49999999999996447 ) ) ;
#40519=APPLICATION_CONTEXT ( 'automotive_design' ) ;
#40952=ORIENTED_EDGE ( 'NONE', *, *, #32286, .T. ) ;
#40954=LINE ( 'NONE', #2498, #96523 ) ;
#40968=CARTESIAN_POINT ( 'NONE',  ( -22.90719435785855751, 144.7012482093458630, 8.500145032286354763E-14 ) ) ;
#41118=LINE ( 'NONE', #27446, #36951 ) ;
#41217=LINE ( 'NONE', #39699, #13355 ) ;
#41347=ORIENTED_EDGE ( 'NONE', *, *, #21213, .F. ) ;
#41407=CARTESIAN_POINT ( 'NONE',  ( 31.94941146435350987, 203.6868197944959320, 22.50000000000001066 ) ) ;
#41431=VECTOR ( 'NONE', #45966, 1000.000000000000114 ) ;
#41433=CARTESIAN_POINT ( 'NONE',  ( -27.52599651137557046, 146.7012482093458914, 1.732050807568941142 ) ) ;
#41545=DIRECTION ( 'NONE',  ( 0.8660254037844384856, 0.5000000000000004441, 0.000000000000000000 ) ) ;
#41739=LINE ( 'NONE', #94993, #87489 ) ;
#41798=EDGE_LOOP ( 'NONE', ( #8168, #3155, #194, #42131, #45928, #61545 ) ) ;
#41962=DIRECTION ( 'NONE',  ( -0.8660254037844384856, -0.5000000000000002220, -3.252519625699449945E-16 ) ) ;
#41992=CARTESIAN_POINT ( 'NONE',  ( -22.42236680055716036, 157.8615022471903444, 5.188172501216621122E-14 ) ) ;
#42131=ORIENTED_EDGE ( 'NONE', *, *, #22404, .T. ) ;
#42265=VECTOR ( 'NONE', #29253, 999.9999999999998863 ) ;
#42267=DIRECTION ( 'NONE',  ( -0.5000000000000001110, 0.8660254037844384856, 0.000000000000000000 ) ) ;
#42475=DIRECTION ( 'NONE',  ( -0.8660254037844384856, -0.5000000000000004441, 0.000000000000000000 ) ) ;
#42914=VECTOR ( 'NONE', #22027, 1000.000000000000000 ) ;
#42973=EDGE_CURVE ( 'NONE', #15205, #85879, #73481, .T. ) ;
#43074=DIRECTION ( 'NONE',  ( -0.8660254037844384856, -0.5000000000000002220, 5.782411586589354927E-17 ) ) ;
#43143=SHAPE_DEFINITION_REPRESENTATION ( #2227, #7571 ) ;
#43280=AXIS2_PLACEMENT_3D ( 'NONE', #21031, #98022, #13424 ) ;
#43324=EDGE_CURVE ( 'NONE', #59740, #5666, #82509, .T. ) ;
#43498=CARTESIAN_POINT ( 'NONE',  ( -26.08262083840154233, 139.2012482093457493, -48.95643923738973768 ) ) ;
#43653=CARTESIAN_POINT ( 'NONE',  ( -19.92236680055716391, 153.5313752282681605, 5.249404841173988696E-14 ) ) ;
#43663=LINE ( 'NONE', #96930, #19772 ) ;
#43674=LINE ( 'NONE', #4181, #81088 ) ;
#43681=EDGE_LOOP ( 'NONE', ( #63779, #69378, #87952, #61663, #83520, #35695, #98437 ) ) ;
#43794=FACE_OUTER_BOUND ( 'NONE', #39555, .T. ) ;
#43803=DIRECTION ( 'NONE',  ( 0.8660254037844383745, 0.5000000000000003331, -0.000000000000000000 ) ) ;
#43846=ORIENTED_EDGE ( 'NONE', *, *, #2048, .F. ) ;
#43986=PLANE ( 'NONE',  #96449 ) ;
#44129=ADVANCED_FACE ( 'NONE', ( #67816 ), #92165, .F. ) ;
#44301=ORIENTED_EDGE ( 'NONE', *, *, #59037, .T. ) ;
#44347=CARTESIAN_POINT ( 'NONE',  ( 28.46864935082047410, 149.7156766241961350, 37.50000000000000000 ) ) ;
#44454=ORIENTED_EDGE ( 'NONE', *, *, #12401, .T. ) ;
#44607=ORIENTED_EDGE ( 'NONE', *, *, #21213, .T. ) ;
#44648=LINE ( 'NONE', #68458, #48988 ) ;
#44655=LINE ( 'NONE', #77064, #6632 ) ;
#44711=CARTESIAN_POINT ( 'NONE',  ( -14.83262083840144996, 124.7156766241961208, 37.49999999999998579 ) ) ;
#44835=ORIENTED_EDGE ( 'NONE', *, *, #4562, .T. ) ;
#45068=ORIENTED_EDGE ( 'NONE', *, *, #65872, .F. ) ;
#45101=LINE ( 'NONE', #27910, #63975 ) ;
#45115=DIRECTION ( 'NONE',  ( -0.5000000000000001110, 0.8660254037844384856, 0.000000000000000000 ) ) ;
#45216=ORIENTED_EDGE ( 'NONE', *, *, #86987, .F. ) ;
#45455=EDGE_LOOP ( 'NONE', ( #93434, #59483 ) ) ;
#45489=DIRECTION ( 'NONE',  ( 0.4999999999999995004, 0.8660254037844389297, 0.000000000000000000 ) ) ;
#45495=CARTESIAN_POINT ( 'NONE',  ( 28.46864935082048831, 149.7156766241961350, -21.50000000000001421 ) ) ;
#45506=DIRECTION ( 'NONE',  ( -0.5000000000000001110, 0.8660254037844384856, 2.775557561562890427E-17 ) ) ;
#45523=DIRECTION ( 'NONE',  ( -2.816764622163176013E-16, -1.626259812849728177E-16, 1.000000000000000000 ) ) ;
#45726=EDGE_CURVE ( 'NONE', #97002, #17498, #117, .T. ) ;
#45768=DIRECTION ( 'NONE',  ( 4.546899780356473057E-16, -0.000000000000000000, -1.000000000000000000 ) ) ;
#45774=EDGE_LOOP ( 'NONE', ( #54386, #23066, #53891, #15311 ) ) ;
#45821=EDGE_CURVE ( 'NONE', #74796, #17687, #57793, .T. ) ;
#45912=LINE ( 'NONE', #76361, #42265 ) ;
#45928=ORIENTED_EDGE ( 'NONE', *, *, #425, .F. ) ;
#45966=DIRECTION ( 'NONE',  ( -0.5000000000000003331, 0.8660254037844383745, -9.251858538542982674E-17 ) ) ;
#46215=LINE ( 'NONE', #36637, #98089 ) ;
#46311=VECTOR ( 'NONE', #41962, 1000.000000000000227 ) ;
#46377=CARTESIAN_POINT ( 'NONE',  ( 28.46864935082050252, 149.7156766241961350, -37.49999999999994316 ) ) ;
#46481=DIRECTION ( 'NONE',  ( 0.7499999999999997780, 0.4330127018922197979, 0.5000000000000000000 ) ) ;
#46921=VECTOR ( 'NONE', #59564, 1000.000000000000000 ) ;
#46934=ORIENTED_EDGE ( 'NONE', *, *, #9947, .F. ) ;
#46983=DIRECTION ( 'NONE',  ( 0.000000000000000000, 1.000000000000000000, -1.090355031989287297E-16 ) ) ;
#47118=FACE_OUTER_BOUND ( 'NONE', #35769, .T. ) ;
#47174=ORIENTED_EDGE ( 'NONE', *, *, #80927, .T. ) ;
#47418=ORIENTED_EDGE ( 'NONE', *, *, #75277, .T. ) ;
#47487=PLANE ( 'NONE',  #71065 ) ;
#47559=VERTEX_POINT ( 'NONE', #7563 ) ;
#47598=VECTOR ( 'NONE', #33846, 1000.000000000000114 ) ;
#47755=VERTEX_POINT ( 'NONE', #41433 ) ;
#47866=PRODUCT_DEFINITION_FORMATION_WITH_SPECIFIED_SOURCE ( 'ANY', '', #29009, .NOT_KNOWN. ) ;
#47877=ORIENTED_EDGE ( 'NONE', *, *, #55877, .T. ) ;
#48072=ORIENTED_EDGE ( 'NONE', *, *, #21324, .F. ) ;
#48124=VECTOR ( 'NONE', #21441, 1000.000000000000114 ) ;
#48277=VECTOR ( 'NONE', #68823, 1000.000000000000000 ) ;
#48296=LINE ( 'NONE', #32591, #98558 ) ;
#48305=ORIENTED_EDGE ( 'NONE', *, *, #85127, .F. ) ;
#48381=FACE_OUTER_BOUND ( 'NONE', #76933, .T. ) ;
#48417=VERTEX_POINT ( 'NONE', #44711 ) ;
#48467=PLANE ( 'NONE',  #10925 ) ;
#48542=CARTESIAN_POINT ( 'NONE',  ( 25.96864935082048831, 154.0458036431183189, 22.50000000000001421 ) ) ;
#48550=ORIENTED_EDGE ( 'NONE', *, *, #17115, .T. ) ;
#48640=CARTESIAN_POINT ( 'NONE',  ( -20.01211276271284945, 173.6868197944959036, 22.50000000000001421 ) ) ;
#48678=ORIENTED_EDGE ( 'NONE', *, *, #30491, .F. ) ;
#48830=VERTEX_POINT ( 'NONE', #7870 ) ;
#48988=VECTOR ( 'NONE', #22365, 1000.000000000000000 ) ;
#49045=CARTESIAN_POINT ( 'NONE',  ( -24.63924516542739696, 141.7012482093459198, 1.426039447152360146E-13 ) ) ;
#49119=EDGE_CURVE ( 'NONE', #83865, #8776, #46215, .T. ) ;
#49348=CARTESIAN_POINT ( 'NONE',  ( 25.96864935082048831, 154.0458036431183189, 30.52142883766506998 ) ) ;
#49426=VERTEX_POINT ( 'NONE', #57825 ) ;
#49513=DIRECTION ( 'NONE',  ( -1.136724945089119250E-16, 1.968865359125295083E-16, 1.000000000000000000 ) ) ;
#49527=VERTEX_POINT ( 'NONE', #39489 ) ;
#49544=DIRECTION ( 'NONE',  ( 1.000000000000000000, 0.000000000000000000, 2.816764622163176999E-16 ) ) ;
#49551=LINE ( 'NONE', #11078, #53784 ) ;
#49559=LINE ( 'NONE', #11087, #46311 ) ;
#49664=LINE ( 'NONE', #51153, #88584 ) ;
#49676=AXIS2_PLACEMENT_3D ( 'NONE', #33779, #81397, #66645 ) ;
#49806=ORIENTED_EDGE ( 'NONE', *, *, #19856, .F. ) ;
#49829=PLANE ( 'NONE',  #91997 ) ;
#50011=CIRCLE ( 'NONE', #11207, 4.999999999999993783 ) ;
#50067=ORIENTED_EDGE ( 'NONE', *, *, #76967, .T. ) ;
#50090=ORIENTED_EDGE ( 'NONE', *, *, #24910, .F. ) ;
#50327=LINE ( 'NONE', #81278, #28535 ) ;
#50443=EDGE_CURVE ( 'NONE', #91009, #72912, #37406, .T. ) ;
#50582=DIRECTION ( 'NONE',  ( 0.5000000000000003331, -0.8660254037844383745, 0.000000000000000000 ) ) ;
#50598=CARTESIAN_POINT ( 'NONE',  ( -26.08262083840154233, 139.2012482093457493, -37.49999999999996447 ) ) ;
#50618=CARTESIAN_POINT ( 'NONE',  ( -27.52599651137551007, 146.7012482093458914, 2.297459087388069147E-14 ) ) ;
#50636=CARTESIAN_POINT ( 'NONE',  ( -21.75249381947929095, 146.7012482093458914, -37.49999999999995737 ) ) ;
#50644=CARTESIAN_POINT ( 'NONE',  ( -0.01211276271276609529, 139.0458036431182620, -21.50000000000001421 ) ) ;
#50702=ORIENTED_EDGE ( 'NONE', *, *, #425, .T. ) ;
#50765=DIRECTION ( 'NONE',  ( 0.8660254037844383745, 0.5000000000000003331, -0.000000000000000000 ) ) ;
#50871=DIRECTION ( 'NONE',  ( 0.8660254037844385966, 0.5000000000000002220, 7.511572993685832627E-16 ) ) ;
#50894=FACE_OUTER_BOUND ( 'NONE', #8478, .T. ) ;
#50988=EDGE_CURVE ( 'NONE', #49426, #85879, #40954, .T. ) ;
#51047=EDGE_LOOP ( 'NONE', ( #58789, #79890 ) ) ;
#51153=CARTESIAN_POINT ( 'NONE',  ( -14.83262083840144996, 124.7156766241961208, 37.49999999999998579 ) ) ;
#51154=ORIENTED_EDGE ( 'NONE', *, *, #22347, .F. ) ;
#51213=PLANE ( 'NONE',  #27285 ) ;
#51240=DIRECTION ( 'NONE',  ( 0.8660254037844383745, 0.5000000000000003331, -0.000000000000000000 ) ) ;
#51251=( NAMED_UNIT ( * ) SI_UNIT ( $, .STERADIAN. ) SOLID_ANGLE_UNIT ( ) );
#51396=MECHANICAL_DESIGN_GEOMETRIC_PRESENTATION_REPRESENTATION('',(#70786),#19036);
#51452=VERTEX_POINT ( 'NONE', #83976 ) ;
#51741=CARTESIAN_POINT ( 'NONE',  ( 28.46864935082048831, 149.7156766241961350, -22.49999999999983658 ) ) ;
#52526=LINE ( 'NONE', #35841, #4388 ) ;
#52528=ORIENTED_EDGE ( 'NONE', *, *, #26131, .F. ) ;
#52630=ORIENTED_EDGE ( 'NONE', *, *, #71134, .T. ) ;
#52661=EDGE_LOOP ( 'NONE', ( #37436, #54286, #96337, #83477, #25091, #25122, #69108, #53890 ) ) ;
#52985=EDGE_CURVE ( 'NONE', #48830, #47755, #3401, .T. ) ;
#53053=CARTESIAN_POINT ( 'NONE',  ( 23.46864935082055226, 158.3759306620404743, 22.50000000000001776 ) ) ;
#53158=EDGE_CURVE ( 'NONE', #77633, #70724, #39718, .T. ) ;
#53170=VECTOR ( 'NONE', #6865, 1000.000000000000000 ) ;
#53507=ORIENTED_EDGE ( 'NONE', *, *, #80927, .F. ) ;
#53784=VECTOR ( 'NONE', #65252, 999.9999999999998863 ) ;
#53793=AXIS2_PLACEMENT_3D ( 'NONE', #29350, #45523, #60214 ) ;
#53881=EDGE_CURVE ( 'NONE', #24841, #83865, #23177, .T. ) ;
#53890=ORIENTED_EDGE ( 'NONE', *, *, #56292, .T. ) ;
#53891=ORIENTED_EDGE ( 'NONE', *, *, #22660, .T. ) ;
#54174=CARTESIAN_POINT ( 'NONE',  ( 5.968649350820482979, 188.6868197944959320, -37.49999999999994316 ) ) ;
#54223=PLANE ( 'NONE',  #58843 ) ;
#54286=ORIENTED_EDGE ( 'NONE', *, *, #94905, .T. ) ;
#54369=ORIENTED_EDGE ( 'NONE', *, *, #32286, .F. ) ;
#54386=ORIENTED_EDGE ( 'NONE', *, *, #43324, .F. ) ;
#54485=VECTOR ( 'NONE', #36284, 1000.000000000000000 ) ;
#54649=EDGE_LOOP ( 'NONE', ( #95058, #15543, #88491, #53507 ) ) ;
#54755=AXIS2_PLACEMENT_3D ( 'NONE', #18479, #27579, #26574 ) ;
#54795=DIRECTION ( 'NONE',  ( 0.8660254037844385966, 0.5000000000000004441, 0.000000000000000000 ) ) ;
#55046=CARTESIAN_POINT ( 'NONE',  ( 19.98788723728717898, 104.4047874917408336, 22.50000000000002132 ) ) ;
#55079=FACE_OUTER_BOUND ( 'NONE', #54649, .T. ) ;
#55369=CARTESIAN_POINT ( 'NONE',  ( 19.98788723728717898, 104.4047874917408336, -22.49999999999983302 ) ) ;
#55426=UNCERTAINTY_MEASURE_WITH_UNIT (LENGTH_MEASURE( 1.000000000000000082E-05 ), #56367, 'distance_accuracy_value', 'NONE');
#55444=VECTOR ( 'NONE', #59796, 1000.000000000000000 ) ;
#55449=CARTESIAN_POINT ( 'NONE',  ( -34.73454462704830803, 165.1868197944959036, 8.171888229646977204E-14 ) ) ;
#55562=LINE ( 'NONE', #25699, #80303 ) ;
#55568=CARTESIAN_POINT ( 'NONE',  ( -35.23882338977090001, 123.3422401859822344, -12.33162903191226789 ) ) ;
#55731=EDGE_LOOP ( 'NONE', ( #35822, #86858, #26394, #79732 ) ) ;
#55877=EDGE_CURVE ( 'NONE', #57299, #83821, #66015, .T. ) ;
#55893=DIRECTION ( 'NONE',  ( -1.850371707708595795E-16, -7.401486830834383181E-16, 1.000000000000000000 ) ) ;
#55958=EDGE_CURVE ( 'NONE', #91009, #47559, #77093, .T. ) ;
#55994=AXIS2_PLACEMENT_3D ( 'NONE', #49348, #96484, #27053 ) ;
#56027=CARTESIAN_POINT ( 'NONE',  ( 23.46864935082055581, 158.3759306620404743, -30.52142883766493853 ) ) ;
#56049=ORIENTED_EDGE ( 'NONE', *, *, #55877, .F. ) ;
#56070=DIRECTION ( 'NONE',  ( 0.8944271909999157444, 0.000000000000000000, -0.4472135954999582608 ) ) ;
#56149=AXIS2_PLACEMENT_3D ( 'NONE', #88114, #18664, #49544 ) ;
#56292=EDGE_CURVE ( 'NONE', #89585, #17687, #25667, .T. ) ;
#56367=( LENGTH_UNIT ( ) NAMED_UNIT ( * ) SI_UNIT ( .MILLI., .METRE. ) );
#56382=AXIS2_PLACEMENT_3D ( 'NONE', #20803, #20298, #95847 ) ;
#56392=CARTESIAN_POINT ( 'NONE',  ( -27.52599651137551007, 146.7012482093458914, -1.732050807568756179 ) ) ;
#56394=AXIS2_PLACEMENT_3D ( 'NONE', #24819, #85689, #87703 ) ;
#56439=ADVANCED_FACE ( 'NONE', ( #89033 ), #19582, .F. ) ;
#56555=FACE_BOUND ( 'NONE', #45455, .T. ) ;
#56930=PLANE ( 'NONE',  #55994 ) ;
#56953=ORIENTED_EDGE ( 'NONE', *, *, #88172, .T. ) ;
#57061=DIRECTION ( 'NONE',  ( 0.5000000000000001110, -0.8660254037844385966, 2.065951763267645480E-16 ) ) ;
#57134=PLANE ( 'NONE',  #56149 ) ;
#57299=VERTEX_POINT ( 'NONE', #68272 ) ;
#57389=CARTESIAN_POINT ( 'NONE',  ( 28.46864935082048831, 149.7156766241961350, 21.50000000000008527 ) ) ;
#57486=EDGE_CURVE ( 'NONE', #83821, #60445, #49664, .T. ) ;
#57682=PLANE ( 'NONE',  #90495 ) ;
#57793=LINE ( 'NONE', #19341, #71982 ) ;
#57825=CARTESIAN_POINT ( 'NONE',  ( 5.968649350820482979, 188.6868197944959320, -37.49999999999994316 ) ) ;
#57864=( NAMED_UNIT ( * ) PLANE_ANGLE_UNIT ( ) SI_UNIT ( $, .RADIAN. ) );
#58135=EDGE_CURVE ( 'NONE', #61485, #17141, #75248, .T. ) ;
#58187=DIRECTION ( 'NONE',  ( 0.8660254037844385966, 0.5000000000000004441, 0.000000000000000000 ) ) ;
#58364=DIRECTION ( 'NONE',  ( -0.5000000000000003331, 0.8660254037844383745, 0.000000000000000000 ) ) ;
#58381=ORIENTED_EDGE ( 'NONE', *, *, #45726, .F. ) ;
#58523=PLANE ( 'NONE',  #21035 ) ;
#58583=FACE_OUTER_BOUND ( 'NONE', #97319, .T. ) ;
#58688=DIRECTION ( 'NONE',  ( 0.8660254037844389297, -0.4999999999999995004, 0.000000000000000000 ) ) ;
#58789=ORIENTED_EDGE ( 'NONE', *, *, #36196, .T. ) ;
#58843=AXIS2_PLACEMENT_3D ( 'NONE', #71469, #1055, #62 ) ;
#58847=DIRECTION ( 'NONE',  ( -0.5000000000000003331, 0.8660254037844383745, -9.251858538542983907E-17 ) ) ;
#58855=EDGE_LOOP ( 'NONE', ( #9889, #25087, #43846, #64929 ) ) ;
#59004=CARTESIAN_POINT ( 'NONE',  ( 28.46864935082048831, 149.7156766241961350, 21.50000000000008527 ) ) ;
#59012=ORIENTED_EDGE ( 'NONE', *, *, #65872, .T. ) ;
#59037=EDGE_CURVE ( 'NONE', #73274, #17687, #98184, .T. ) ;
#59063=ADVANCED_FACE ( 'NONE', ( #13577 ), #28765, .F. ) ;
#59483=ORIENTED_EDGE ( 'NONE', *, *, #77639, .F. ) ;
#59489=EDGE_CURVE ( 'NONE', #47559, #77633, #50327, .T. ) ;
#59494=VECTOR ( 'NONE', #14434, 1000.000000000000114 ) ;
#59564=DIRECTION ( 'NONE',  ( -8.673617379884075901E-16, 0.000000000000000000, 1.000000000000000000 ) ) ;
#59740=VERTEX_POINT ( 'NONE', #78130 ) ;
#59755=FACE_OUTER_BOUND ( 'NONE', #20510, .T. ) ;
#59796=DIRECTION ( 'NONE',  ( -0.4999999999999995004, 0.8660254037844389297, -1.249000902703319567E-14 ) ) ;
#59856=ORIENTED_EDGE ( 'NONE', *, *, #31778, .F. ) ;
#59922=LINE ( 'NONE', #92370, #48124 ) ;
#60214=DIRECTION ( 'NONE',  ( 1.000000000000000000, 0.000000000000000000, 2.816764622163176013E-16 ) ) ;
#60247=EDGE_LOOP ( 'NONE', ( #32452, #10434, #20423, #92227 ) ) ;
#60445=VERTEX_POINT ( 'NONE', #89240 ) ;
#60640=ORIENTED_EDGE ( 'NONE', *, *, #14029, .F. ) ;
#61097=ORIENTED_EDGE ( 'NONE', *, *, #85127, .T. ) ;
#61485=VERTEX_POINT ( 'NONE', #23237 ) ;
#61517=ADVANCED_FACE ( 'NONE', ( #77963 ), #38936, .F. ) ;
#61545=ORIENTED_EDGE ( 'NONE', *, *, #25834, .F. ) ;
#61663=ORIENTED_EDGE ( 'NONE', *, *, #69840, .F. ) ;
#61711=ADVANCED_FACE ( 'NONE', ( #81004 ), #57134, .F. ) ;
#61819=EDGE_CURVE ( 'NONE', #16529, #82623, #52526, .T. ) ;
#61860=VERTEX_POINT ( 'NONE', #98164 ) ;
#61955=CARTESIAN_POINT ( 'NONE',  ( -27.52599651137550651, 146.7012482093459198, -37.49999999999995737 ) ) ;
#62075=EDGE_LOOP ( 'NONE', ( #48678, #30769, #73363, #25369, #21288, #47877, #64878 ) ) ;
#62227=LINE ( 'NONE', #31831, #33638 ) ;
#62245=ORIENTED_EDGE ( 'NONE', *, *, #58135, .T. ) ;
#62357=AXIS2_PLACEMENT_3D ( 'NONE', #54174, #85143, #15689 ) ;
#62373=CARTESIAN_POINT ( 'NONE',  ( -19.83262083840137180, 133.3759306620404459, -30.52142883766495629 ) ) ;
#62385=CARTESIAN_POINT ( 'NONE',  ( 42.87900647455834502, 24.75620593066997444, -1.732050807568748407 ) ) ;
#62504=VECTOR ( 'NONE', #83004, 1000.000000000000000 ) ;
#62534=DIRECTION ( 'NONE',  ( 0.4330127018922195758, 0.2500000000000004441, 0.8660254037844384856 ) ) ;
#62674=DIRECTION ( 'NONE',  ( 0.4472135954999574836, 0.7745966692414836263, 0.4472135954999578722 ) ) ;
#62771=EDGE_CURVE ( 'NONE', #89587, #73274, #95679, .T. ) ;
#62901=AXIS2_PLACEMENT_3D ( 'NONE', #87944, #27083, #17990 ) ;
#62931=( NAMED_UNIT ( * ) PLANE_ANGLE_UNIT ( ) SI_UNIT ( $, .RADIAN. ) );
#62952=DIRECTION ( 'NONE',  ( -0.5000000000000003331, 0.8660254037844383745, 0.000000000000000000 ) ) ;
#63251=AXIS2_PLACEMENT_3D ( 'NONE', #68146, #82423, #67153 ) ;
#63259=DIRECTION ( 'NONE',  ( 8.673617379884076887E-16, 0.000000000000000000, -1.000000000000000000 ) ) ;
#63295=CARTESIAN_POINT ( 'NONE',  ( -37.33262083840145351, 163.6868197944958467, 37.49999999999998579 ) ) ;
#63546=CARTESIAN_POINT ( 'NONE',  ( -17.33262083840142509, 129.0458036431182904, -21.50000000000003197 ) ) ;
#63672=VERTEX_POINT ( 'NONE', #2969 ) ;
#63695=DIRECTION ( 'NONE',  ( 0.4330127018922195758, 0.2500000000000004441, 0.8660254037844384856 ) ) ;
#63766=VERTEX_POINT ( 'NONE', #48542 ) ;
#63779=ORIENTED_EDGE ( 'NONE', *, *, #12401, .F. ) ;
#63975=VECTOR ( 'NONE', #20833, 1000.000000000000000 ) ;
#64054=DIRECTION ( 'NONE',  ( -0.000000000000000000, -0.000000000000000000, 1.000000000000000000 ) ) ;
#64130=ADVANCED_FACE ( 'NONE', ( #43794 ), #11930, .F. ) ;
#64176=ORIENTED_EDGE ( 'NONE', *, *, #71134, .F. ) ;
#64198=VECTOR ( 'NONE', #26539, 1000.000000000000000 ) ;
#64233=CARTESIAN_POINT ( 'NONE',  ( 25.96864935082050252, 154.0458036431183189, -30.52142883766499892 ) ) ;
#64241=CARTESIAN_POINT ( 'NONE',  ( -14.83262083840142154, 124.7156766241961208, -37.49999999999995737 ) ) ;
#64371=VECTOR ( 'NONE', #76314, 1000.000000000000227 ) ;
#64494=DIRECTION ( 'NONE',  ( 4.336808689942034499E-16, 7.511572993685835585E-16, -1.000000000000000000 ) ) ;
#64615=CARTESIAN_POINT ( 'NONE',  ( 25.96864935082050252, 154.0458036431183189, -21.50000000000001421 ) ) ;
#64685=EDGE_LOOP ( 'NONE', ( #86921, #17929, #30424, #14688 ) ) ;
#64719=DIRECTION ( 'NONE',  ( 0.000000000000000000, 1.000000000000000000, -1.090355031989287297E-16 ) ) ;
#64878=ORIENTED_EDGE ( 'NONE', *, *, #57486, .T. ) ;
#64929=ORIENTED_EDGE ( 'NONE', *, *, #50443, .F. ) ;
#64992=ORIENTED_EDGE ( 'NONE', *, *, #19629, .T. ) ;
#65170=VECTOR ( 'NONE', #28459, 1000.000000000000227 ) ;
#65232=DIRECTION ( 'NONE',  ( 0.8660254037844384856, 0.5000000000000002220, -5.782411586589354927E-17 ) ) ;
#65252=DIRECTION ( 'NONE',  ( 0.5000000000000002220, -0.8660254037844385966, 9.251858538542986372E-17 ) ) ;
#65405=DIRECTION ( 'NONE',  ( 0.5000000000000002220, -0.8660254037844385966, 9.251858538542986372E-17 ) ) ;
#65493=DIRECTION ( 'NONE',  ( -1.850371707708595795E-16, -7.401486830834383181E-16, 1.000000000000000000 ) ) ;
#65578=CARTESIAN_POINT ( 'NONE',  ( 42.87900647455834502, 24.75620593066997444, 8.404119662683931360E-14 ) ) ;
#65612=DIRECTION ( 'NONE',  ( -0.5000000000000003331, 0.8660254037844383745, 0.000000000000000000 ) ) ;
#65623=VERTEX_POINT ( 'NONE', #18571 ) ;
#65792=CIRCLE ( 'NONE', #94997, 4.999999999999993783 ) ;
#65872=EDGE_CURVE ( 'NONE', #72912, #8322, #81473, .T. ) ;
#65912=CARTESIAN_POINT ( 'NONE',  ( -38.63165894407827494, 162.9368197944959036, 2.598076211353396392 ) ) ;
#65967=PRODUCT_CONTEXT ( 'NONE', #29179, 'mechanical' ) ;
#65974=CYLINDRICAL_SURFACE ( 'NONE', #19520, 4.999999999999993783 ) ;
#66015=LINE ( 'NONE', #87405, #14037 ) ;
#66027=CARTESIAN_POINT ( 'NONE',  ( -13.79761285583127872, 128.9229902121449811, 8.559299291603829198E-14 ) ) ;
#66139=VECTOR ( 'NONE', #95183, 1000.000000000000227 ) ;
#66645=DIRECTION ( 'NONE',  ( -0.8660254037844384856, -0.5000000000000002220, 0.000000000000000000 ) ) ;
#66741=CARTESIAN_POINT ( 'NONE',  ( 25.96864935082048831, 154.0458036431183189, 21.50000000000008527 ) ) ;
#66957=CARTESIAN_POINT ( 'NONE',  ( 25.96864935082050252, 154.0458036431183189, -30.52142883766499892 ) ) ;
#66969=ORIENTED_EDGE ( 'NONE', *, *, #18849, .F. ) ;
#67153=DIRECTION ( 'NONE',  ( -0.5000000000000001110, 0.8660254037844384856, 0.000000000000000000 ) ) ;
#67283=CARTESIAN_POINT ( 'NONE',  ( 71.94941146435354540, 134.4047874917408478, -22.49999999999983658 ) ) ;
#67291=DIRECTION ( 'NONE',  ( -0.5000000000000003331, 0.8660254037844383745, -9.251858538542983907E-17 ) ) ;
#67380=ORIENTED_EDGE ( 'NONE', *, *, #36196, .F. ) ;
#67391=CARTESIAN_POINT ( 'NONE',  ( 25.96864935082048831, 154.0458036431183189, 22.50000000000001421 ) ) ;
#67462=VECTOR ( 'NONE', #31983, 1000.000000000000000 ) ;
#67619=ORIENTED_EDGE ( 'NONE', *, *, #75277, .F. ) ;
#67713=DIRECTION ( 'NONE',  ( 0.8660254037844385966, 0.5000000000000002220, 7.511572993685832627E-16 ) ) ;
#67816=FACE_OUTER_BOUND ( 'NONE', #41798, .T. ) ;
#68146=CARTESIAN_POINT ( 'NONE',  ( 42.87900647455834502, 24.75620593066997444, 8.404119662683931360E-14 ) ) ;
#68162=CARTESIAN_POINT ( 'NONE',  ( -21.75249381947928740, 146.7012482093458914, 37.49999999999996447 ) ) ;
#68272=CARTESIAN_POINT ( 'NONE',  ( 5.968649350820469657, 188.6868197944958752, 37.50000000000000000 ) ) ;
#68458=CARTESIAN_POINT ( 'NONE',  ( -19.83262083840137180, 133.3759306620404459, -30.52142883766495629 ) ) ;
#68539=LINE ( 'NONE', #30040, #38561 ) ;
#68700=ADVANCED_FACE ( 'NONE', ( #85403 ), #93493, .F. ) ;
#68707=ADVANCED_FACE ( 'NONE', ( #32147 ), #8363, .F. ) ;
#68784=AXIS2_PLACEMENT_3D ( 'NONE', #15354, #91924, #23457 ) ;
#68823=DIRECTION ( 'NONE',  ( -0.000000000000000000, -0.000000000000000000, 1.000000000000000000 ) ) ;
#68889=ORIENTED_EDGE ( 'NONE', *, *, #70740, .T. ) ;
#68910=LINE ( 'NONE', #51741, #98463 ) ;
#69108=ORIENTED_EDGE ( 'NONE', *, *, #20676, .T. ) ;
#69147=EDGE_LOOP ( 'NONE', ( #26667, #2098, #64176, #17920, #91435, #4062, #45068 ) ) ;
#69248=CARTESIAN_POINT ( 'NONE',  ( -13.79761285583127872, 128.9229902121449811, 8.559299291603829198E-14 ) ) ;
#69378=ORIENTED_EDGE ( 'NONE', *, *, #879, .T. ) ;
#69379=ADVANCED_BREP_SHAPE_REPRESENTATION ( '', ( #76056, #68784 ), #31602 ) ;
#69698=ORIENTED_EDGE ( 'NONE', *, *, #21324, .T. ) ;
#69815=VECTOR ( 'NONE', #555, 1000.000000000000000 ) ;
#69840=EDGE_CURVE ( 'NONE', #15205, #97002, #96783, .T. ) ;
#69938=LINE ( 'NONE', #86709, #69815 ) ;
#70387=ORIENTED_EDGE ( 'NONE', *, *, #93410, .F. ) ;
#70395=PLANE ( 'NONE',  #62357 ) ;
#70686=CARTESIAN_POINT ( 'NONE',  ( -24.63924516542737919, 141.7012482093459766, -37.49999999999996447 ) ) ;
#70695=LINE ( 'NONE', #46377, #7006 ) ;
#70724=VERTEX_POINT ( 'NONE', #28332 ) ;
#70740=EDGE_CURVE ( 'NONE', #74234, #21771, #76452, .T. ) ;
#70786=STYLED_ITEM('',(#100338),#76056);
#70880=ORIENTED_EDGE ( 'NONE', *, *, #33162, .T. ) ;
#70913=EDGE_CURVE ( 'NONE', #71581, #21771, #90456, .T. ) ;
#70920=AXIS2_PLACEMENT_3D ( 'NONE', #750, #62534, #24052 ) ;
#71015=EDGE_CURVE ( 'NONE', #74234, #77633, #29112, .T. ) ;
#71065=AXIS2_PLACEMENT_3D ( 'NONE', #94631, #63695, #56070 ) ;
#71106=CARTESIAN_POINT ( 'NONE',  ( 23.46864935082055581, 158.3759306620404743, -30.52142883766493853 ) ) ;
#71134=EDGE_CURVE ( 'NONE', #4349, #8776, #48296, .T. ) ;
#71355=ORIENTED_EDGE ( 'NONE', *, *, #55958, .T. ) ;
#71447=CARTESIAN_POINT ( 'NONE',  ( 86.18027666378029039, 49.75620593066999220, -22.49999999999982592 ) ) ;
#71469=CARTESIAN_POINT ( 'NONE',  ( 71.94941146435354540, 134.4047874917408478, 22.50000000000001776 ) ) ;
#71578=ADVANCED_FACE ( 'NONE', ( #55079 ), #47487, .F. ) ;
#71581=VERTEX_POINT ( 'NONE', #8993 ) ;
#71701=CARTESIAN_POINT ( 'NONE',  ( -0.01211276271276783001, 139.0458036431182620, 22.50000000000001776 ) ) ;
#71733=ORIENTED_EDGE ( 'NONE', *, *, #71828, .F. ) ;
#71828=EDGE_CURVE ( 'NONE', #17141, #17498, #33176, .T. ) ;
#71899=EDGE_LOOP ( 'NONE', ( #11363, #67619, #19049, #10634 ) ) ;
#71965=DIRECTION ( 'NONE',  ( 0.8944271909999156334, 0.000000000000000000, -0.4472135954999582053 ) ) ;
#71982=VECTOR ( 'NONE', #65405, 999.9999999999998863 ) ;
#72457=VECTOR ( 'NONE', #10240, 1000.000000000000227 ) ;
#72623=DIRECTION ( 'NONE',  ( -0.5000000000000003331, 0.8660254037844383745, -9.251858538542983907E-17 ) ) ;
#72912=VERTEX_POINT ( 'NONE', #88967 ) ;
#72929=DIRECTION ( 'NONE',  ( -0.5000000000000003331, 0.8660254037844383745, 0.000000000000000000 ) ) ;
#73238=CARTESIAN_POINT ( 'NONE',  ( -2.512112762712737091, 143.3759306620403891, 22.50000000000002132 ) ) ;
#73274=VERTEX_POINT ( 'NONE', #73238 ) ;
#73363=ORIENTED_EDGE ( 'NONE', *, *, #92492, .T. ) ;
#73414=DIRECTION ( 'NONE',  ( -0.5000000000000001110, 0.8660254037844384856, 0.000000000000000000 ) ) ;
#73481=LINE ( 'NONE', #4065, #99320 ) ;
#73502=FACE_OUTER_BOUND ( 'NONE', #64685, .T. ) ;
#73707=ORIENTED_EDGE ( 'NONE', *, *, #16908, .T. ) ;
#73746=CARTESIAN_POINT ( 'NONE',  ( 28.46864935082047410, 149.7156766241961350, 37.50000000000000000 ) ) ;
#73788=CARTESIAN_POINT ( 'NONE',  ( -17.33262083840143930, 129.0458036431182904, 30.52142883766505221 ) ) ;
#73969=CARTESIAN_POINT ( 'NONE',  ( -24.92236680055716036, 162.1916292661125283, 5.188172501216621122E-14 ) ) ;
#74022=ADVANCED_FACE ( 'NONE', ( #34733 ), #58523, .F. ) ;
#74234=VERTEX_POINT ( 'NONE', #33120 ) ;
#74280=CARTESIAN_POINT ( 'NONE',  ( 25.96864935082048831, 154.0458036431183189, 30.52142883766506998 ) ) ;
#74426=CARTESIAN_POINT ( 'NONE',  ( 86.18027666378027618, 49.75620593066998509, 1.003037947553365612E-13 ) ) ;
#74638=VERTEX_POINT ( 'NONE', #98312 ) ;
#74796=VERTEX_POINT ( 'NONE', #18131 ) ;
#74989=ORIENTED_EDGE ( 'NONE', *, *, #23936, .T. ) ;
#75079=SHAPE_REPRESENTATION_RELATIONSHIP ( 'NONE' , 'NONE' ,  #7571, #69379 ) ;
#75088=CARTESIAN_POINT ( 'NONE',  ( -0.01211276271276956473, 139.0458036431182620, 21.50000000000008527 ) ) ;
#75136=DIRECTION ( 'NONE',  ( 0.4330127018922192983, 0.2500000000000001110, -0.8660254037844387076 ) ) ;
#75150=ADVANCED_FACE ( 'NONE', ( #18903 ), #65974, .F. ) ;
#75248=LINE ( 'NONE', #6329, #59494 ) ;
#75251=VECTOR ( 'NONE', #24845, 1000.000000000000227 ) ;
#75277=EDGE_CURVE ( 'NONE', #7578, #59740, #22361, .T. ) ;
#75789=DIRECTION ( 'NONE',  ( -0.5000000000000003331, 0.8660254037844383745, 0.000000000000000000 ) ) ;
#76056=MANIFOLD_SOLID_BREP ( 'Cut-Extrude16', #2199 ) ;
#76135=VECTOR ( 'NONE', #38037, 1000.000000000000000 ) ;
#76179=DIRECTION ( 'NONE',  ( -1.000000000000000000, 0.000000000000000000, 0.000000000000000000 ) ) ;
#76314=DIRECTION ( 'NONE',  ( -0.8660254037844384856, -0.5000000000000002220, -3.252519625699449945E-16 ) ) ;
#76327=FACE_OUTER_BOUND ( 'NONE', #52661, .T. ) ;
#76361=CARTESIAN_POINT ( 'NONE',  ( 86.18027666378029039, 49.75620593066999220, -22.49999999999982592 ) ) ;
#76452=LINE ( 'NONE', #21737, #48277 ) ;
#76579=DIRECTION ( 'NONE',  ( -0.5000000000000008882, 0.8660254037844381525, 0.000000000000000000 ) ) ;
#76611=CARTESIAN_POINT ( 'NONE',  ( -22.42236680055716036, 157.8615022471903444, 5.188172501216621122E-14 ) ) ;
#76733=ORIENTED_EDGE ( 'NONE', *, *, #22040, .F. ) ;
#76816=AXIS2_PLACEMENT_3D ( 'NONE', #14515, #67713, #7916 ) ;
#76933=EDGE_LOOP ( 'NONE', ( #27277, #88492, #29059, #83642 ) ) ;
#76967=EDGE_CURVE ( 'NONE', #27862, #63672, #4014, .T. ) ;
#77064=CARTESIAN_POINT ( 'NONE',  ( -14.83262083840143575, 124.7156766241961208, 21.50000000000006750 ) ) ;
#77093=LINE ( 'NONE', #62373, #67462 ) ;
#77100=DIRECTION ( 'NONE',  ( -0.5000000000000003331, 0.8660254037844383745, 0.000000000000000000 ) ) ;
#77189=EDGE_CURVE ( 'NONE', #20145, #8322, #29314, .T. ) ;
#77303=CARTESIAN_POINT ( 'NONE',  ( 28.46864935082047410, 149.7156766241961350, 37.50000000000000000 ) ) ;
#77489=ORIENTED_EDGE ( 'NONE', *, *, #81793, .T. ) ;
#77521=AXIS2_PLACEMENT_3D ( 'NONE', #3574, #41545, #4548 ) ;
#77633=VERTEX_POINT ( 'NONE', #7251 ) ;
#77639=EDGE_CURVE ( 'NONE', #32226, #27140, #22320, .T. ) ;
#77774=PRODUCT_DEFINITION_CONTEXT ( 'detailed design', #40519, 'design' ) ;
#77776=DIRECTION ( 'NONE',  ( 0.8660254037844384856, 0.5000000000000002220, 0.000000000000000000 ) ) ;
#77963=FACE_OUTER_BOUND ( 'NONE', #43681, .T. ) ;
#78039=PLANE ( 'NONE',  #56394 ) ;
#78063=FACE_OUTER_BOUND ( 'NONE', #3325, .T. ) ;
#78130=CARTESIAN_POINT ( 'NONE',  ( -0.01211276271276956473, 139.0458036431182620, 21.50000000000006750 ) ) ;
#78131=VECTOR ( 'NONE', #62674, 1000.000000000000000 ) ;
#78150=CARTESIAN_POINT ( 'NONE',  ( -17.33262083840143930, 129.0458036431182904, 21.50000000000006750 ) ) ;
#78316=DIRECTION ( 'NONE',  ( -0.8660254037844384856, -0.5000000000000002220, -3.252519625699449945E-16 ) ) ;
#78378=DIRECTION ( 'NONE',  ( -0.8660254037844384856, -0.5000000000000004441, 0.000000000000000000 ) ) ;
#78409=LINE ( 'NONE', #55568, #78131 ) ;
#78415=CARTESIAN_POINT ( 'NONE',  ( -17.23454462704816947, 134.8759306620403038, 8.444826468009708598E-14 ) ) ;
#79121=ADVANCED_FACE ( 'NONE', ( #73502 ), #28377, .F. ) ;
#79325=PLANE ( 'NONE',  #62901 ) ;
#79469=LINE ( 'NONE', #79963, #39264 ) ;
#79470=LINE ( 'NONE', #41407, #47598 ) ;
#79551=DIRECTION ( 'NONE',  ( -1.850371707708595795E-16, -7.401486830834383181E-16, 1.000000000000000000 ) ) ;
#79666=CARTESIAN_POINT ( 'NONE',  ( 28.46864935082047410, 149.7156766241961350, 37.50000000000000000 ) ) ;
#79732=ORIENTED_EDGE ( 'NONE', *, *, #52985, .F. ) ;
#79754=CARTESIAN_POINT ( 'NONE',  ( -24.63924516542741827, 141.7012482093459198, 37.49999999999996447 ) ) ;
#79766=ADVANCED_FACE ( 'NONE', ( #12162 ), #97285, .T. ) ;
#79860=ORIENTED_EDGE ( 'NONE', *, *, #2646, .T. ) ;
#79890=ORIENTED_EDGE ( 'NONE', *, *, #24910, .T. ) ;
#79963=CARTESIAN_POINT ( 'NONE',  ( -21.13165894407813994, 132.6259306620403322, 2.598076211353400833 ) ) ;
#79981=VECTOR ( 'NONE', #21741, 1000.000000000000000 ) ;
#80010=PRODUCT_DEFINITION ( 'UNKNOWN', '', #47866, #77774 ) ;
#80171=LINE ( 'NONE', #65912, #20793 ) ;
#80224=CIRCLE ( 'NONE', #97976, 4.999999999999993783 ) ;
#80233=VECTOR ( 'NONE', #81520, 1000.000000000000114 ) ;
#80240=ORIENTED_EDGE ( 'NONE', *, *, #24594, .T. ) ;
#80244=DIRECTION ( 'NONE',  ( 8.673617379884080832E-16, -0.000000000000000000, -1.000000000000000000 ) ) ;
#80303=VECTOR ( 'NONE', #32278, 1000.000000000000227 ) ;
#80411=CARTESIAN_POINT ( 'NONE',  ( -19.83262083840135759, 133.3759306620403891, -1.732050807568708217 ) ) ;
#80672=VECTOR ( 'NONE', #28808, 1000.000000000000000 ) ;
#80716=CARTESIAN_POINT ( 'NONE',  ( -19.92236680055716391, 153.5313752282681605, 5.249404841173988696E-14 ) ) ;
#80927=EDGE_CURVE ( 'NONE', #8776, #51452, #81016, .T. ) ;
#80991=DIRECTION ( 'NONE',  ( 4.336808689942034499E-16, 7.511572993685835585E-16, -1.000000000000000000 ) ) ;
#81004=FACE_OUTER_BOUND ( 'NONE', #13774, .T. ) ;
#81016=LINE ( 'NONE', #11080, #29066 ) ;
#81088=VECTOR ( 'NONE', #34109, 1000.000000000000000 ) ;
#81278=CARTESIAN_POINT ( 'NONE',  ( -17.33262083840142509, 129.0458036431182904, -30.52142883766501669 ) ) ;
#81299=ORIENTED_EDGE ( 'NONE', *, *, #53158, .T. ) ;
#81309=FACE_OUTER_BOUND ( 'NONE', #33017, .T. ) ;
#81397=DIRECTION ( 'NONE',  ( -0.5000000000000003331, 0.8660254037844385966, -2.273449890178237515E-16 ) ) ;
#81409=LINE ( 'NONE', #44347, #6186 ) ;
#81458=DIRECTION ( 'NONE',  ( -0.7499999999999995559, -0.4330127018922196314, 0.5000000000000004441 ) ) ;
#81473=LINE ( 'NONE', #49045, #19240 ) ;
#81499=DIRECTION ( 'NONE',  ( 0.5000000000000001110, -0.8660254037844385966, 2.065951763267645480E-16 ) ) ;
#81520=DIRECTION ( 'NONE',  ( 0.4999999999999987788, -0.8660254037844392627, -0.000000000000000000 ) ) ;
#81532=FACE_OUTER_BOUND ( 'NONE', #71899, .T. ) ;
#81606=DIRECTION ( 'NONE',  ( -0.5000000000000002220, 0.8660254037844385966, 0.000000000000000000 ) ) ;
#81630=AXIS2_PLACEMENT_3D ( 'NONE', #45495, #28304, #22209 ) ;
#81729=ORIENTED_EDGE ( 'NONE', *, *, #94905, .F. ) ;
#81759=VERTEX_POINT ( 'NONE', #73969 ) ;
#81793=EDGE_CURVE ( 'NONE', #49527, #71581, #4553, .T. ) ;
#81949=EDGE_LOOP ( 'NONE', ( #52630, #47174, #89164, #29488, #35825, #21895, #49806, #9934 ) ) ;
#81987=VECTOR ( 'NONE', #45506, 1000.000000000000227 ) ;
#82423=DIRECTION ( 'NONE',  ( 0.8660254037844385966, 0.5000000000000002220, 7.511572993685832627E-16 ) ) ;
#82509=LINE ( 'NONE', #66741, #36239 ) ;
#82623=VERTEX_POINT ( 'NONE', #48640 ) ;
#82679=CARTESIAN_POINT ( 'NONE',  ( 23.46864935082044923, 158.3759306620404459, 22.50000000000001776 ) ) ;
#82682=FACE_OUTER_BOUND ( 'NONE', #81949, .T. ) ;
#82885=VERTEX_POINT ( 'NONE', #73788 ) ;
#82900=EDGE_LOOP ( 'NONE', ( #71733, #37065, #97696, #56049, #81729, #17430, #9460, #76733, #21094, #28505, #2564 ) ) ;
#82999=ORIENTED_EDGE ( 'NONE', *, *, #16908, .F. ) ;
#83004=DIRECTION ( 'NONE',  ( 0.8660254037844384856, 0.5000000000000002220, -5.782411586589354927E-17 ) ) ;
#83136=CARTESIAN_POINT ( 'NONE',  ( 28.46864935082048831, 149.7156766241961350, -22.49999999999984013 ) ) ;
#83159=DIRECTION ( 'NONE',  ( 0.8660254037844385966, 0.5000000000000002220, 7.511572993685832627E-16 ) ) ;
#83477=ORIENTED_EDGE ( 'NONE', *, *, #94948, .T. ) ;
#83520=ORIENTED_EDGE ( 'NONE', *, *, #96045, .T. ) ;
#83535=CARTESIAN_POINT ( 'NONE',  ( -19.83262083840140022, 133.3759306620404459, 30.52142883766498827 ) ) ;
#83642=ORIENTED_EDGE ( 'NONE', *, *, #59037, .F. ) ;
#83758=VECTOR ( 'NONE', #49513, 1000.000000000000000 ) ;
#83787=DIRECTION ( 'NONE',  ( -0.4472135954999574281, -0.7745966692414834043, 0.4472135954999583718 ) ) ;
#83821=VERTEX_POINT ( 'NONE', #63295 ) ;
#83865=VERTEX_POINT ( 'NONE', #40968 ) ;
#83914=CARTESIAN_POINT ( 'NONE',  ( -24.63924516542738274, 141.7012482093459198, 1.732050807568909834 ) ) ;
#83918=CARTESIAN_POINT ( 'NONE',  ( 2.487887237287232711, 134.7156766241960497, -21.50000000000001421 ) ) ;
#83976=CARTESIAN_POINT ( 'NONE',  ( -19.83262083840137180, 133.3759306620403891, 1.732050807568888073 ) ) ;
#84057=VECTOR ( 'NONE', #35453, 1000.000000000000000 ) ;
#84144=EDGE_CURVE ( 'NONE', #20145, #38493, #41739, .T. ) ;
#84226=ORIENTED_EDGE ( 'NONE', *, *, #5582, .T. ) ;
#84553=ADVANCED_FACE ( 'NONE', ( #30146 ), #37247, .F. ) ;
#84934=ORIENTED_EDGE ( 'NONE', *, *, #2646, .F. ) ;
#85127=EDGE_CURVE ( 'NONE', #89587, #16529, #24983, .T. ) ;
#85143=DIRECTION ( 'NONE',  ( 0.5000000000000003331, -0.8660254037844385966, -5.484689767424254197E-16 ) ) ;
#85209=EDGE_CURVE ( 'NONE', #4349, #38493, #43674, .T. ) ;
#85316=EDGE_CURVE ( 'NONE', #92799, #5666, #44655, .T. ) ;
#85403=FACE_OUTER_BOUND ( 'NONE', #31750, .T. ) ;
#85607=ORIENTED_EDGE ( 'NONE', *, *, #22347, .T. ) ;
#85689=DIRECTION ( 'NONE',  ( -0.8660254037844384856, -0.5000000000000004441, 0.000000000000000000 ) ) ;
#85806=EDGE_CURVE ( 'NONE', #31218, #21771, #45912, .T. ) ;
#85879=VERTEX_POINT ( 'NONE', #86370 ) ;
#86227=ORIENTED_EDGE ( 'NONE', *, *, #71828, .T. ) ;
#86370=CARTESIAN_POINT ( 'NONE',  ( -37.33262083840143930, 163.6868197944959036, -37.49999999999995737 ) ) ;
#86513=DIRECTION ( 'NONE',  ( 4.546899780356473057E-16, -0.000000000000000000, -1.000000000000000000 ) ) ;
#86709=CARTESIAN_POINT ( 'NONE',  ( 23.46864935082055581, 158.3759306620404743, -22.49999999999984013 ) ) ;
#86824=VECTOR ( 'NONE', #63259, 1000.000000000000000 ) ;
#86838=VERTEX_POINT ( 'NONE', #43653 ) ;
#86858=ORIENTED_EDGE ( 'NONE', *, *, #58135, .F. ) ;
#86918=ORIENTED_EDGE ( 'NONE', *, *, #57486, .F. ) ;
#86921=ORIENTED_EDGE ( 'NONE', *, *, #69840, .T. ) ;
#86987=EDGE_CURVE ( 'NONE', #61860, #89587, #69938, .T. ) ;
#87000=ORIENTED_EDGE ( 'NONE', *, *, #55958, .F. ) ;
#87069=CARTESIAN_POINT ( 'NONE',  ( 28.46864935082048831, 149.7156766241961350, 22.50000000000001776 ) ) ;
#87224=ORIENTED_EDGE ( 'NONE', *, *, #85806, .F. ) ;
#87232=CARTESIAN_POINT ( 'NONE',  ( -24.92236680055716036, 162.1916292661125283, 5.188172501216621122E-14 ) ) ;
#87311=LINE ( 'NONE', #2647, #72457 ) ;
#87386=EDGE_LOOP ( 'NONE', ( #87224, #100011, #27753, #80240, #60640, #56953, #84226, #68889 ) ) ;
#87405=CARTESIAN_POINT ( 'NONE',  ( 5.968649350820469657, 188.6868197944958752, 37.50000000000000000 ) ) ;
#87422=ORIENTED_EDGE ( 'NONE', *, *, #50988, .F. ) ;
#87489=VECTOR ( 'NONE', #27060, 1000.000000000000000 ) ;
#87703=DIRECTION ( 'NONE',  ( 0.5000000000000003331, -0.8660254037844383745, 0.000000000000000000 ) ) ;
#87888=ORIENTED_EDGE ( 'NONE', *, *, #98974, .F. ) ;
#87906=ORIENTED_EDGE ( 'NONE', *, *, #91374, .T. ) ;
#87944=CARTESIAN_POINT ( 'NONE',  ( 71.94941146435354540, 134.4047874917408478, 22.50000000000001776 ) ) ;
#87952=ORIENTED_EDGE ( 'NONE', *, *, #31778, .T. ) ;
#87963=ORIENTED_EDGE ( 'NONE', *, *, #43324, .T. ) ;
#88011=DIRECTION ( 'NONE',  ( 2.816764622163176999E-16, 1.626259812849726452E-16, -1.000000000000000000 ) ) ;
#88114=CARTESIAN_POINT ( 'NONE',  ( 28.46864935082050252, 149.7156766241961350, -37.49999999999994316 ) ) ;
#88172=EDGE_CURVE ( 'NONE', #61860, #6163, #92427, .T. ) ;
#88359=VERTEX_POINT ( 'NONE', #27500 ) ;
#88491=ORIENTED_EDGE ( 'NONE', *, *, #93410, .T. ) ;
#88492=ORIENTED_EDGE ( 'NONE', *, *, #98473, .T. ) ;
#88494=ORIENTED_EDGE ( 'NONE', *, *, #86987, .T. ) ;
#88499=ORIENTED_EDGE ( 'NONE', *, *, #23936, .F. ) ;
#88584=VECTOR ( 'NONE', #12690, 1000.000000000000114 ) ;
#88665=DIRECTION ( 'NONE',  ( 0.8660254037844385966, 0.5000000000000002220, 7.511572993685832627E-16 ) ) ;
#88822=EDGE_CURVE ( 'NONE', #89585, #18415, #62227, .T. ) ;
#88967=CARTESIAN_POINT ( 'NONE',  ( -24.63924516542738274, 141.7012482093459198, -1.732050807568746853 ) ) ;
#88984=DIRECTION ( 'NONE',  ( 0.5000000000000003331, -0.8660254037844385966, 0.000000000000000000 ) ) ;
#89000=CARTESIAN_POINT ( 'NONE',  ( -22.42236680055716036, 157.8615022471903444, 5.188172501216621122E-14 ) ) ;
#89033=FACE_OUTER_BOUND ( 'NONE', #21615, .T. ) ;
#89116=CARTESIAN_POINT ( 'NONE',  ( 23.46864935082055581, 158.3759306620404743, -30.52142883766493853 ) ) ;
#89164=ORIENTED_EDGE ( 'NONE', *, *, #1639, .F. ) ;
#89170=CARTESIAN_POINT ( 'NONE',  ( 19.98788723728717898, 104.4047874917408336, 22.50000000000002132 ) ) ;
#89240=CARTESIAN_POINT ( 'NONE',  ( -27.52599651137547809, 146.7012482093459198, 37.49999999999998579 ) ) ;
#89245=DIRECTION ( 'NONE',  ( -0.8660254037844384856, -0.5000000000000002220, 0.000000000000000000 ) ) ;
#89557=CARTESIAN_POINT ( 'NONE',  ( 71.94941146435354540, 134.4047874917408478, -22.49999999999983658 ) ) ;
#89585=VERTEX_POINT ( 'NONE', #99897 ) ;
#89587=VERTEX_POINT ( 'NONE', #7683 ) ;
#89848=VERTEX_POINT ( 'NONE', #908 ) ;
#89862=DIRECTION ( 'NONE',  ( -0.8944271909999158554, 0.000000000000000000, -0.4472135954999578722 ) ) ;
#89866=ORIENTED_EDGE ( 'NONE', *, *, #96045, .F. ) ;
#89954=FACE_OUTER_BOUND ( 'NONE', #33895, .T. ) ;
#90026=CARTESIAN_POINT ( 'NONE',  ( -27.52599651137551007, 146.7012482093458914, 2.297459087388069147E-14 ) ) ;
#90032=LINE ( 'NONE', #28689, #54485 ) ;
#90135=PLANE ( 'NONE',  #22038 ) ;
#90349=VERTEX_POINT ( 'NONE', #26429 ) ;
#90354=VECTOR ( 'NONE', #96253, 1000.000000000000000 ) ;
#90456=LINE ( 'NONE', #36187, #93730 ) ;
#90495=AXIS2_PLACEMENT_3D ( 'NONE', #89170, #42475, #50582 ) ;
#90628=EDGE_CURVE ( 'NONE', #85879, #17498, #94460, .T. ) ;
#91004=ADVANCED_FACE ( 'NONE', ( #56555, #95621 ), #48467, .F. ) ;
#91009=VERTEX_POINT ( 'NONE', #80411 ) ;
#91374=EDGE_CURVE ( 'NONE', #63672, #7578, #24785, .T. ) ;
#91435=ORIENTED_EDGE ( 'NONE', *, *, #84144, .F. ) ;
#91496=CARTESIAN_POINT ( 'NONE',  ( -13.76211276271278194, 162.8615022471903444, 5.188172501216621122E-14 ) ) ;
#91670=ORIENTED_EDGE ( 'NONE', *, *, #38764, .F. ) ;
#91730=VECTOR ( 'NONE', #86513, 1000.000000000000000 ) ;
#91924=DIRECTION ( 'NONE',  ( 0.000000000000000000, 0.000000000000000000, 1.000000000000000000 ) ) ;
#91997=AXIS2_PLACEMENT_3D ( 'NONE', #66027, #75136, #89862 ) ;
#92150=CARTESIAN_POINT ( 'NONE',  ( 19.98788723728717898, 104.4047874917408336, -22.49999999999983302 ) ) ;
#92165=PLANE ( 'NONE',  #81630 ) ;
#92227=ORIENTED_EDGE ( 'NONE', *, *, #9947, .T. ) ;
#92370=CARTESIAN_POINT ( 'NONE',  ( 2.487887237287232711, 134.7156766241960497, -21.50000000000002487 ) ) ;
#92427=LINE ( 'NONE', #71106, #9975 ) ;
#92492=EDGE_CURVE ( 'NONE', #4349, #48417, #41217, .T. ) ;
#92656=CARTESIAN_POINT ( 'NONE',  ( 42.87900647455834502, 24.75620593066997444, -1.732050807568748407 ) ) ;
#92799=VERTEX_POINT ( 'NONE', #3633 ) ;
#92833=ORIENTED_EDGE ( 'NONE', *, *, #71015, .F. ) ;
#93180=DIRECTION ( 'NONE',  ( 0.000000000000000000, 1.000000000000000000, 0.000000000000000000 ) ) ;
#93410=EDGE_CURVE ( 'NONE', #24841, #51452, #79469, .T. ) ;
#93434=ORIENTED_EDGE ( 'NONE', *, *, #17115, .F. ) ;
#93493=PLANE ( 'NONE',  #19380 ) ;
#93730=VECTOR ( 'NONE', #65232, 1000.000000000000000 ) ;
#94192=ORIENTED_EDGE ( 'NONE', *, *, #42973, .T. ) ;
#94238=ORIENTED_EDGE ( 'NONE', *, *, #52985, .T. ) ;
#94460=LINE ( 'NONE', #17419, #33707 ) ;
#94502=VECTOR ( 'NONE', #46481, 1000.000000000000000 ) ;
#94631=CARTESIAN_POINT ( 'NONE',  ( -17.69472717286124208, 126.6729902121449811, 2.598076211353400389 ) ) ;
#94887=AXIS2_PLACEMENT_3D ( 'NONE', #69248, #100176, #14064 ) ;
#94892=DIRECTION ( 'NONE',  ( 0.8660254037844385966, 0.5000000000000004441, 0.000000000000000000 ) ) ;
#94905=EDGE_CURVE ( 'NONE', #74796, #57299, #10811, .T. ) ;
#94948=EDGE_CURVE ( 'NONE', #14526, #16186, #33609, .T. ) ;
#94993=CARTESIAN_POINT ( 'NONE',  ( -21.75249381947928740, 146.7012482093458914, -48.95643923738973768 ) ) ;
#94997=AXIS2_PLACEMENT_3D ( 'NONE', #91496, #23037, #75789 ) ;
#95058=ORIENTED_EDGE ( 'NONE', *, *, #49119, .F. ) ;
#95183=DIRECTION ( 'NONE',  ( -0.8660254037844384856, -0.5000000000000002220, -3.252519625699449945E-16 ) ) ;
#95202=AXIS2_PLACEMENT_3D ( 'NONE', #95420, #94892, #62952 ) ;
#95383=LINE ( 'NONE', #79666, #3041 ) ;
#95392=DIRECTION ( 'NONE',  ( 0.7499999999999991118, 0.4330127018922202420, -0.5000000000000004441 ) ) ;
#95420=CARTESIAN_POINT ( 'NONE',  ( -13.76211276271278194, 162.8615022471903444, 5.188172501216621122E-14 ) ) ;
#95509=FACE_OUTER_BOUND ( 'NONE', #60247, .T. ) ;
#95621=FACE_OUTER_BOUND ( 'NONE', #99291, .T. ) ;
#95679=LINE ( 'NONE', #18634, #83758 ) ;
#95847=DIRECTION ( 'NONE',  ( -0.5000000000000001110, 0.8660254037844384856, 0.000000000000000000 ) ) ;
#95977=LINE ( 'NONE', #17422, #64198 ) ;
#96045=EDGE_CURVE ( 'NONE', #15205, #20145, #12669, .T. ) ;
#96253=DIRECTION ( 'NONE',  ( -2.168404344971022180E-16, 3.755786496842918286E-16, 1.000000000000000000 ) ) ;
#96261=CARTESIAN_POINT ( 'NONE',  ( 25.96864935082048831, 154.0458036431183189, 30.52142883766506998 ) ) ;
#96337=ORIENTED_EDGE ( 'NONE', *, *, #35737, .T. ) ;
#96429=VECTOR ( 'NONE', #43074, 1000.000000000000000 ) ;
#96449=AXIS2_PLACEMENT_3D ( 'NONE', #43498, #58688, #45489 ) ;
#96484=DIRECTION ( 'NONE',  ( -6.526680975732919234E-15, 1.065403912962273439E-14, 1.000000000000000000 ) ) ;
#96502=EDGE_CURVE ( 'NONE', #59740, #27862, #26128, .T. ) ;
#96523=VECTOR ( 'NONE', #25799, 1000.000000000000227 ) ;
#96620=CARTESIAN_POINT ( 'NONE',  ( 42.87900647455834502, 24.75620593066997444, 1.732050807568941364 ) ) ;
#96783=LINE ( 'NONE', #50618, #7854 ) ;
#96930=CARTESIAN_POINT ( 'NONE',  ( 19.98788723728717898, 104.4047874917408336, 22.50000000000002132 ) ) ;
#96964=DIRECTION ( 'NONE',  ( -0.8660254037844384856, -0.5000000000000002220, -3.252519625699449945E-16 ) ) ;
#96988=CARTESIAN_POINT ( 'NONE',  ( 2.487887237287232711, 134.7156766241960497, 21.50000000000007461 ) ) ;
#97002=VERTEX_POINT ( 'NONE', #56392 ) ;
#97285=PLANE ( 'NONE',  #77521 ) ;
#97319=EDGE_LOOP ( 'NONE', ( #9045, #26902, #48305, #45216 ) ) ;
#97327=LINE ( 'NONE', #67391, #96429 ) ;
#97394=LINE ( 'NONE', #66957, #65170 ) ;
#97696=ORIENTED_EDGE ( 'NONE', *, *, #26131, .T. ) ;
#97729=FACE_OUTER_BOUND ( 'NONE', #69147, .T. ) ;
#97976=AXIS2_PLACEMENT_3D ( 'NONE', #76611, #54795, #77100 ) ;
#97990=FACE_OUTER_BOUND ( 'NONE', #8670, .T. ) ;
#98022=DIRECTION ( 'NONE',  ( -5.963328051300290638E-15, 1.097929109219269329E-14, -1.000000000000000000 ) ) ;
#98089=VECTOR ( 'NONE', #83787, 999.9999999999998863 ) ;
#98125=ORIENTED_EDGE ( 'NONE', *, *, #98974, .T. ) ;
#98164=CARTESIAN_POINT ( 'NONE',  ( 23.46864935082046344, 158.3759306620404743, -22.49999999999983658 ) ) ;
#98184=LINE ( 'NONE', #53053, #62504 ) ;
#98289=CARTESIAN_POINT ( 'NONE',  ( 28.46864935082048831, 149.7156766241961350, 21.50000000000008527 ) ) ;
#98293=ORIENTED_EDGE ( 'NONE', *, *, #81793, .F. ) ;
#98312=CARTESIAN_POINT ( 'NONE',  ( 28.46864935082050252, 149.7156766241961350, -37.49999999999994316 ) ) ;
#98371=AXIS2_PLACEMENT_3D ( 'NONE', #89557, #34308, #64719 ) ;
#98437=ORIENTED_EDGE ( 'NONE', *, *, #30491, .T. ) ;
#98463=VECTOR ( 'NONE', #99835, 1000.000000000000000 ) ;
#98473=EDGE_CURVE ( 'NONE', #82623, #74796, #79470, .T. ) ;
#98558=VECTOR ( 'NONE', #64494, 1000.000000000000000 ) ;
#98679=ADVANCED_FACE ( 'NONE', ( #76327 ), #29708, .T. ) ;
#98974=EDGE_CURVE ( 'NONE', #81759, #27140, #4047, .T. ) ;
#99291=EDGE_LOOP ( 'NONE', ( #61097, #24966, #33124, #36351 ) ) ;
#99320=VECTOR ( 'NONE', #81606, 999.9999999999998863 ) ;
#99467=LINE ( 'NONE', #40504, #25425 ) ;
#99835=DIRECTION ( 'NONE',  ( -0.8660254037844384856, -0.5000000000000002220, 5.782411586589354927E-17 ) ) ;
#99897=CARTESIAN_POINT ( 'NONE',  ( 23.46864935082052739, 158.3759306620404743, 30.52142883766500603 ) ) ;
#99924=LINE ( 'NONE', #8212, #17537 ) ;
#100011=ORIENTED_EDGE ( 'NONE', *, *, #25834, .T. ) ;
#100176=DIRECTION ( 'NONE',  ( 0.4330127018922192983, 0.2500000000000001110, -0.8660254037844387076 ) ) ;
#100268=DIRECTION ( 'NONE',  ( 0.000000000000000000, -0.000000000000000000, 1.000000000000000000 ) ) ;
#100332=COLOUR_RGB('Black',0.12,0.14,0.17);
#100333=FILL_AREA_STYLE_COLOUR('',#100332);
#100334=FILL_AREA_STYLE('',(#100333));
#100335=SURFACE_STYLE_FILL_AREA(#100334);
#100336=SURFACE_SIDE_STYLE('',(#100335));
#100337=SURFACE_STYLE_USAGE(.BOTH.,#100336);
#100338=PRESENTATION_STYLE_ASSIGNMENT((#100337));
ENDSEC;
END-ISO-10303-21;
